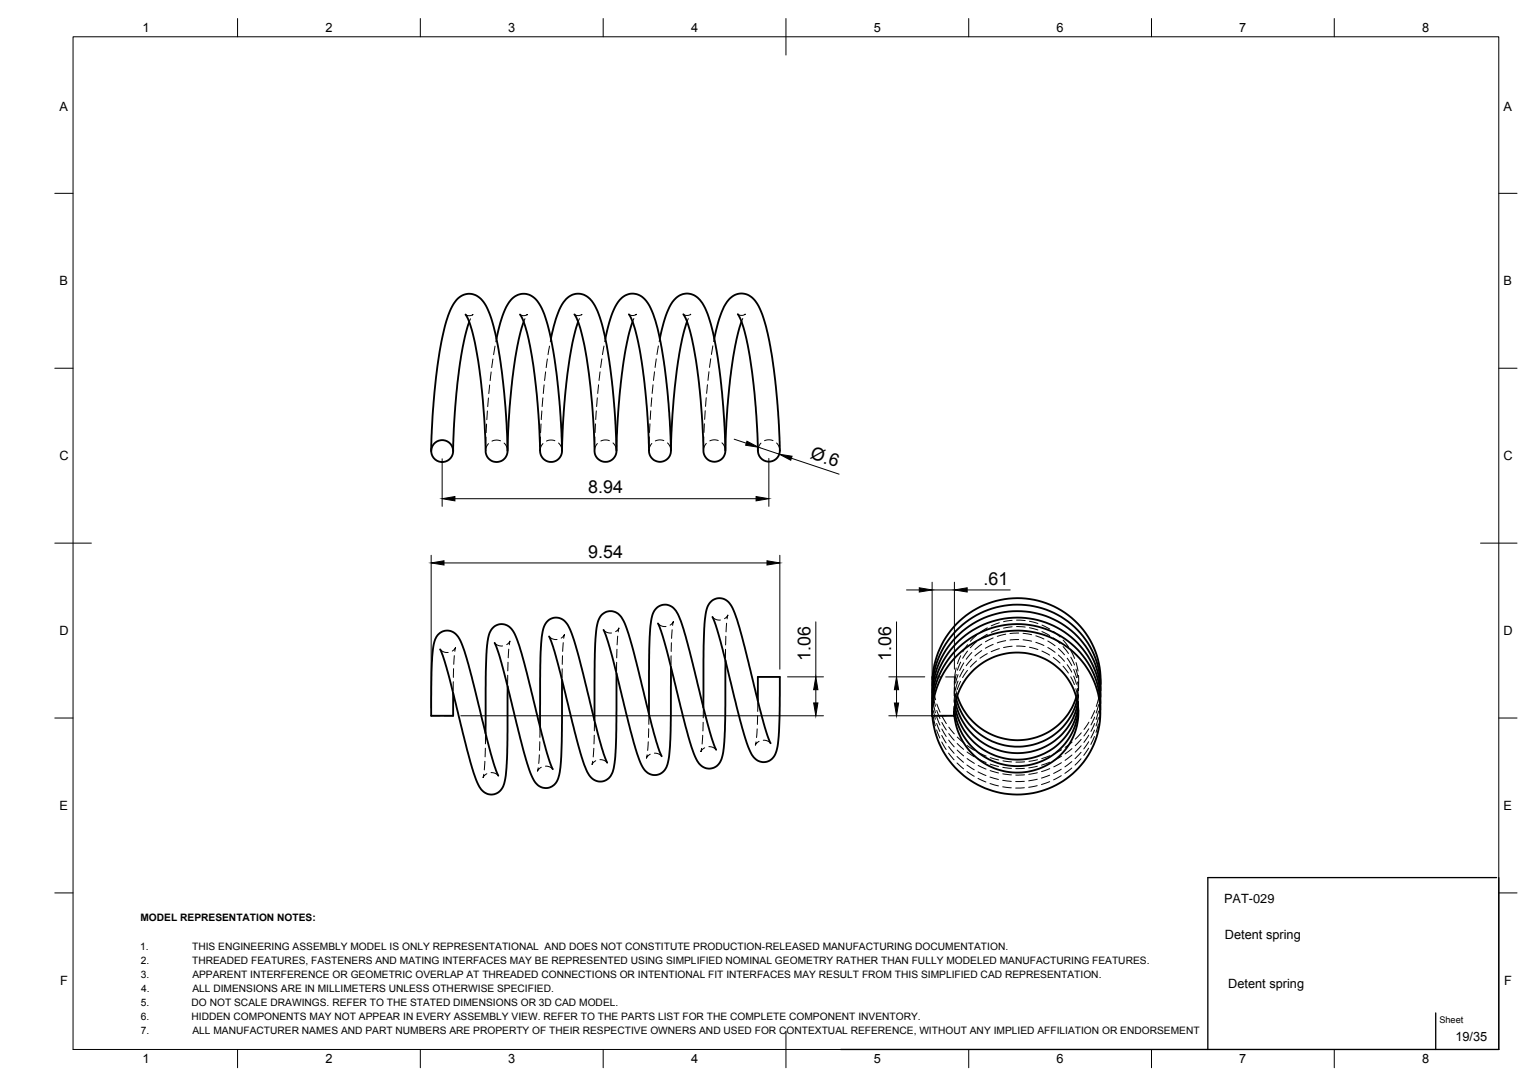
ISO-10303-21;
HEADER;
/* Generated by software containing ST-Developer
 * from STEP Tools, Inc. (www.steptools.com) 
 */

FILE_DESCRIPTION(
/* description */ ('Door-style hinge test fixture with detent'),
/* implementation_level */ '2;1');

FILE_NAME(
/* name */ 'Detent spring.step',
/* time_stamp */ '2026-10-28T03:24:57-07:00',
/* author */ (''),
/* organization */ (''),
/* preprocessor_version */ 'ST-DEVELOPER v20.2',
/* originating_system */ 'Autodesk Translation Framework v15.17.0.0',
/* authorisation */ '');

FILE_SCHEMA (('AUTOMOTIVE_DESIGN { 1 0 10303 214 3 1 1 }'));
ENDSEC;

DATA;
#10=MECHANICAL_DESIGN_GEOMETRIC_PRESENTATION_REPRESENTATION('',(#337),#9813);
#221=B_SPLINE_CURVE_WITH_KNOTS('',3,(#8567,#8568,#8569,#8570,#8571,#8572,
#8573,#8574,#8575,#8576,#8577,#8578,#8579,#8580,#8581,#8582,#8583,#8584,
#8585,#8586,#8587,#8588,#8589,#8590,#8591,#8592,#8593,#8594,#8595,#8596,
#8597,#8598,#8599,#8600,#8601,#8602,#8603,#8604,#8605,#8606,#8607,#8608,
#8609,#8610,#8611,#8612,#8613,#8614,#8615,#8616,#8617,#8618,#8619,#8620,
#8621,#8622,#8623,#8624,#8625,#8626,#8627,#8628,#8629,#8630,#8631),
 .UNSPECIFIED.,.F.,.F.,(4,1,1,1,1,1,1,1,1,1,1,1,1,1,1,1,1,1,1,1,1,1,1,1,
1,1,1,1,1,1,1,1,1,1,1,1,1,1,1,1,1,1,1,1,1,1,1,1,1,1,1,1,1,1,1,1,1,1,1,1,
1,1,4),(0.,0.0178571428571429,0.0357142857142857,0.0535714285714286,0.0714285714285714,
0.0892857142857143,0.107142857142857,0.125,0.142857142857143,0.158730158730159,
0.174603174603175,0.19047619047619,0.202380952380952,0.214285714285714,
0.226190476190476,0.238095238095238,0.25,0.261904761904762,0.273809523809524,
0.285714285714286,0.30952380952381,0.333333333333333,0.357142857142857,
0.380952380952381,0.404761904761905,0.428571428571429,0.446428571428571,
0.464285714285714,0.482142857142857,0.5,0.508928571428571,0.517857142857143,
0.535714285714286,0.553571428571429,0.571428571428571,0.589285714285714,
0.607142857142857,0.625,0.642857142857143,0.660714285714286,0.678571428571428,
0.696428571428571,0.714285714285714,0.738095238095238,0.75,0.761904761904762,
0.773809523809524,0.785714285714286,0.797619047619047,0.809523809523809,
0.821428571428571,0.833333333333333,0.845238095238095,0.857142857142857,
0.866071428571429,0.875,0.892857142857143,0.910714285714286,0.928571428571429,
0.946428571428571,0.964285714285714,0.982142857142857,1.),.UNSPECIFIED.);
#241=B_SPLINE_SURFACE_WITH_KNOTS('',3,3,((#7914,#7915,#7916,#7917,#7918,
#7919,#7920,#7921,#7922,#7923,#7924,#7925,#7926,#7927,#7928,#7929,#7930,
#7931,#7932,#7933,#7934,#7935,#7936,#7937,#7938,#7939,#7940,#7941,#7942,
#7943,#7944,#7945,#7946,#7947,#7948,#7949,#7950,#7951,#7952,#7953,#7954,
#7955,#7956,#7957,#7958,#7959,#7960,#7961,#7962,#7963,#7964,#7965,#7966,
#7967,#7968,#7969,#7970,#7971,#7972,#7973,#7974,#7975,#7976,#7977,#7978),
(#7979,#7980,#7981,#7982,#7983,#7984,#7985,#7986,#7987,#7988,#7989,#7990,
#7991,#7992,#7993,#7994,#7995,#7996,#7997,#7998,#7999,#8000,#8001,#8002,
#8003,#8004,#8005,#8006,#8007,#8008,#8009,#8010,#8011,#8012,#8013,#8014,
#8015,#8016,#8017,#8018,#8019,#8020,#8021,#8022,#8023,#8024,#8025,#8026,
#8027,#8028,#8029,#8030,#8031,#8032,#8033,#8034,#8035,#8036,#8037,#8038,
#8039,#8040,#8041,#8042,#8043),(#8044,#8045,#8046,#8047,#8048,#8049,#8050,
#8051,#8052,#8053,#8054,#8055,#8056,#8057,#8058,#8059,#8060,#8061,#8062,
#8063,#8064,#8065,#8066,#8067,#8068,#8069,#8070,#8071,#8072,#8073,#8074,
#8075,#8076,#8077,#8078,#8079,#8080,#8081,#8082,#8083,#8084,#8085,#8086,
#8087,#8088,#8089,#8090,#8091,#8092,#8093,#8094,#8095,#8096,#8097,#8098,
#8099,#8100,#8101,#8102,#8103,#8104,#8105,#8106,#8107,#8108),(#8109,#8110,
#8111,#8112,#8113,#8114,#8115,#8116,#8117,#8118,#8119,#8120,#8121,#8122,
#8123,#8124,#8125,#8126,#8127,#8128,#8129,#8130,#8131,#8132,#8133,#8134,
#8135,#8136,#8137,#8138,#8139,#8140,#8141,#8142,#8143,#8144,#8145,#8146,
#8147,#8148,#8149,#8150,#8151,#8152,#8153,#8154,#8155,#8156,#8157,#8158,
#8159,#8160,#8161,#8162,#8163,#8164,#8165,#8166,#8167,#8168,#8169,#8170,
#8171,#8172,#8173),(#8174,#8175,#8176,#8177,#8178,#8179,#8180,#8181,#8182,
#8183,#8184,#8185,#8186,#8187,#8188,#8189,#8190,#8191,#8192,#8193,#8194,
#8195,#8196,#8197,#8198,#8199,#8200,#8201,#8202,#8203,#8204,#8205,#8206,
#8207,#8208,#8209,#8210,#8211,#8212,#8213,#8214,#8215,#8216,#8217,#8218,
#8219,#8220,#8221,#8222,#8223,#8224,#8225,#8226,#8227,#8228,#8229,#8230,
#8231,#8232,#8233,#8234,#8235,#8236,#8237,#8238),(#8239,#8240,#8241,#8242,
#8243,#8244,#8245,#8246,#8247,#8248,#8249,#8250,#8251,#8252,#8253,#8254,
#8255,#8256,#8257,#8258,#8259,#8260,#8261,#8262,#8263,#8264,#8265,#8266,
#8267,#8268,#8269,#8270,#8271,#8272,#8273,#8274,#8275,#8276,#8277,#8278,
#8279,#8280,#8281,#8282,#8283,#8284,#8285,#8286,#8287,#8288,#8289,#8290,
#8291,#8292,#8293,#8294,#8295,#8296,#8297,#8298,#8299,#8300,#8301,#8302,
#8303),(#8304,#8305,#8306,#8307,#8308,#8309,#8310,#8311,#8312,#8313,#8314,
#8315,#8316,#8317,#8318,#8319,#8320,#8321,#8322,#8323,#8324,#8325,#8326,
#8327,#8328,#8329,#8330,#8331,#8332,#8333,#8334,#8335,#8336,#8337,#8338,
#8339,#8340,#8341,#8342,#8343,#8344,#8345,#8346,#8347,#8348,#8349,#8350,
#8351,#8352,#8353,#8354,#8355,#8356,#8357,#8358,#8359,#8360,#8361,#8362,
#8363,#8364,#8365,#8366,#8367,#8368),(#8369,#8370,#8371,#8372,#8373,#8374,
#8375,#8376,#8377,#8378,#8379,#8380,#8381,#8382,#8383,#8384,#8385,#8386,
#8387,#8388,#8389,#8390,#8391,#8392,#8393,#8394,#8395,#8396,#8397,#8398,
#8399,#8400,#8401,#8402,#8403,#8404,#8405,#8406,#8407,#8408,#8409,#8410,
#8411,#8412,#8413,#8414,#8415,#8416,#8417,#8418,#8419,#8420,#8421,#8422,
#8423,#8424,#8425,#8426,#8427,#8428,#8429,#8430,#8431,#8432,#8433),(#8434,
#8435,#8436,#8437,#8438,#8439,#8440,#8441,#8442,#8443,#8444,#8445,#8446,
#8447,#8448,#8449,#8450,#8451,#8452,#8453,#8454,#8455,#8456,#8457,#8458,
#8459,#8460,#8461,#8462,#8463,#8464,#8465,#8466,#8467,#8468,#8469,#8470,
#8471,#8472,#8473,#8474,#8475,#8476,#8477,#8478,#8479,#8480,#8481,#8482,
#8483,#8484,#8485,#8486,#8487,#8488,#8489,#8490,#8491,#8492,#8493,#8494,
#8495,#8496,#8497,#8498),(#8499,#8500,#8501,#8502,#8503,#8504,#8505,#8506,
#8507,#8508,#8509,#8510,#8511,#8512,#8513,#8514,#8515,#8516,#8517,#8518,
#8519,#8520,#8521,#8522,#8523,#8524,#8525,#8526,#8527,#8528,#8529,#8530,
#8531,#8532,#8533,#8534,#8535,#8536,#8537,#8538,#8539,#8540,#8541,#8542,
#8543,#8544,#8545,#8546,#8547,#8548,#8549,#8550,#8551,#8552,#8553,#8554,
#8555,#8556,#8557,#8558,#8559,#8560,#8561,#8562,#8563)),.UNSPECIFIED.,.T.,
 .F.,.F.,(4,1,1,1,1,1,1,4),(4,1,1,1,1,1,1,1,1,1,1,1,1,1,1,1,1,1,1,1,1,1,
1,1,1,1,1,1,1,1,1,1,1,1,1,1,1,1,1,1,1,1,1,1,1,1,1,1,1,1,1,1,1,1,1,1,1,1,
1,1,1,1,4),(-3.14159265358979,-2.24399475256414,-1.34639685153848,-0.448798950512828,
0.448798950512828,1.34639685153848,2.24399475256414,3.14159265358979),(0.,
0.0178571428571429,0.0357142857142857,0.0535714285714286,0.0714285714285714,
0.0892857142857143,0.107142857142857,0.125,0.142857142857143,0.158730158730159,
0.174603174603175,0.19047619047619,0.202380952380952,0.214285714285714,
0.226190476190476,0.238095238095238,0.25,0.261904761904762,0.273809523809524,
0.285714285714286,0.30952380952381,0.333333333333333,0.357142857142857,
0.380952380952381,0.404761904761905,0.428571428571429,0.446428571428571,
0.464285714285714,0.482142857142857,0.5,0.508928571428571,0.517857142857143,
0.535714285714286,0.553571428571429,0.571428571428571,0.589285714285714,
0.607142857142857,0.625,0.642857142857143,0.660714285714286,0.678571428571428,
0.696428571428571,0.714285714285714,0.738095238095238,0.75,0.761904761904762,
0.773809523809524,0.785714285714286,0.797619047619047,0.809523809523809,
0.821428571428571,0.833333333333333,0.845238095238095,0.857142857142857,
0.866071428571429,0.875,0.892857142857143,0.910714285714286,0.928571428571429,
0.946428571428571,0.964285714285714,0.982142857142857,1.),.UNSPECIFIED.);
#274=SHAPE_REPRESENTATION_RELATIONSHIP('SRR','None',#9951,#305);
#305=ADVANCED_BREP_SHAPE_REPRESENTATION('',(#377),#9794);
#337=STYLED_ITEM('',(#10183),#377);
#377=MANIFOLD_SOLID_BREP('Body1',#4768);
#578=PLANE('',#5393);
#579=PLANE('',#5394);
#790=FACE_OUTER_BOUND('',#1141,.T.);
#791=FACE_OUTER_BOUND('',#1142,.T.);
#792=FACE_OUTER_BOUND('',#1143,.T.);
#1141=EDGE_LOOP('',(#3773,#3774,#3775,#3776));
#1142=EDGE_LOOP('',(#3777));
#1143=EDGE_LOOP('',(#3778));
#2083=CIRCLE('',#5391,0.03);
#2084=CIRCLE('',#5392,0.03);
#2411=VERTEX_POINT('',#8564);
#2412=VERTEX_POINT('',#8566);
#2903=EDGE_CURVE('',#2411,#2411,#2083,.T.);
#2904=EDGE_CURVE('',#2411,#2412,#221,.T.);
#2905=EDGE_CURVE('',#2412,#2412,#2084,.T.);
#3773=ORIENTED_EDGE('',*,*,#2903,.T.);
#3774=ORIENTED_EDGE('',*,*,#2904,.T.);
#3775=ORIENTED_EDGE('',*,*,#2905,.F.);
#3776=ORIENTED_EDGE('',*,*,#2904,.F.);
#3777=ORIENTED_EDGE('',*,*,#2905,.T.);
#3778=ORIENTED_EDGE('',*,*,#2903,.F.);
#4595=ADVANCED_FACE('',(#790),#241,.T.);
#4596=ADVANCED_FACE('',(#791),#578,.T.);
#4597=ADVANCED_FACE('',(#792),#579,.F.);
#4768=CLOSED_SHELL('',(#4595,#4596,#4597));
#5390=AXIS2_PLACEMENT_3D('',#7913,#6429,#6430);
#5391=AXIS2_PLACEMENT_3D('',#8565,#6431,#6432);
#5392=AXIS2_PLACEMENT_3D('',#8632,#6433,#6434);
#5393=AXIS2_PLACEMENT_3D('',#8633,#6435,#6436);
#5394=AXIS2_PLACEMENT_3D('',#8634,#6437,#6438);
#6429=DIRECTION('axis',(0.,0.,1.));
#6430=DIRECTION('refdir',(1.,0.,0.));
#6431=DIRECTION('center_axis',(-0.000133970394124395,-0.118176177591672,
0.992992634968536));
#6432=DIRECTION('ref_axis',(1.59438332031483E-5,-0.992992644005897,-0.118176176516135));
#6433=DIRECTION('center_axis',(0.000133970209996934,-0.118176177452328,
0.992992634985144));
#6434=DIRECTION('ref_axis',(0.970349186816215,0.240028974349624,0.0284349629466645));
#6435=DIRECTION('center_axis',(0.000133970209996934,-0.118176177452328,
0.992992634985144));
#6436=DIRECTION('ref_axis',(0.970349186816215,0.240028974349624,0.0284349629466645));
#6437=DIRECTION('center_axis',(-0.000133970394124395,-0.118176177591672,
0.992992634968536));
#6438=DIRECTION('ref_axis',(1.59438332031483E-5,-0.992992644005897,-0.118176176516135));
#7913=CARTESIAN_POINT('',(0.,0.,0.));
#7914=CARTESIAN_POINT('Ctrl Pts',(0.199999521685004,-2.62021022067982,7.20354528529548));
#7915=CARTESIAN_POINT('Ctrl Pts',(0.19999343949118,-2.6255753643916,7.24862669087077));
#7916=CARTESIAN_POINT('Ctrl Pts',(0.168615691452697,-2.63634781999191,7.33868016798294));
#7917=CARTESIAN_POINT('Ctrl Pts',(0.0459616996448183,-2.65270477799173,
7.41618164971903));
#7918=CARTESIAN_POINT('Ctrl Pts',(-0.0998469869656992,-2.66924595959392,
7.39996507729611));
#7919=CARTESIAN_POINT('Ctrl Pts',(-0.204936181985623,-2.68597304189578,
7.29527847685269));
#7920=CARTESIAN_POINT('Ctrl Pts',(-0.221986969755699,-2.7028797483455,7.14628505326925));
#7921=CARTESIAN_POINT('Ctrl Pts',(-0.141631327334848,-2.71996166380803,
7.01788664502262));
#7922=CARTESIAN_POINT('Ctrl Pts',(0.00270481241442627,-2.73721192504324,
6.96708134679183));
#7923=CARTESIAN_POINT('Ctrl Pts',(0.143039113459417,-2.75397833948373,7.01603761180454));
#7924=CARTESIAN_POINT('Ctrl Pts',(0.223330027417085,-2.77023316539608,7.13370506584288));
#7925=CARTESIAN_POINT('Ctrl Pts',(0.223609433092684,-2.7859516486779,7.2713911725354));
#7926=CARTESIAN_POINT('Ctrl Pts',(0.152101468687107,-2.80045790761646,7.37648984952004));
#7927=CARTESIAN_POINT('Ctrl Pts',(0.0493840180807327,-2.81371750007274,
7.42583309513969));
#7928=CARTESIAN_POINT('Ctrl Pts',(-0.0535656424988985,-2.82570326133932,
7.42596307871198));
#7929=CARTESIAN_POINT('Ctrl Pts',(-0.146731811694293,-2.83773755003964,
7.38108373553243));
#7930=CARTESIAN_POINT('Ctrl Pts',(-0.211512387655128,-2.8498166397957,7.29998894076038));
#7931=CARTESIAN_POINT('Ctrl Pts',(-0.234672692510252,-2.86193666288461,
7.19851881716116));
#7932=CARTESIAN_POINT('Ctrl Pts',(-0.211502078818359,-2.87409363541626,
7.09651570260184));
#7933=CARTESIAN_POINT('Ctrl Pts',(-0.146175031667225,-2.88628349462379,
7.01496045942807));
#7934=CARTESIAN_POINT('Ctrl Pts',(-0.0201759406699065,-2.90257490033143,
6.95334279019282));
#7935=CARTESIAN_POINT('Ctrl Pts',(0.164048433167981,-2.92300029227989,6.99488705015939));
#7936=CARTESIAN_POINT('Ctrl Pts',(0.263212640482471,-2.94757377707087,7.20034626829039));
#7937=CARTESIAN_POINT('Ctrl Pts',(0.16413428164115,-2.9721746956776,7.40571604889496));
#7938=CARTESIAN_POINT('Ctrl Pts',(-0.0580809020736254,-2.99676718133414,
7.45651943873815));
#7939=CARTESIAN_POINT('Ctrl Pts',(-0.236127517621773,-3.02131545740765,
7.31427023254914));
#7940=CARTESIAN_POINT('Ctrl Pts',(-0.235623291843773,-3.04374517395574,
7.10674242176483));
#7941=CARTESIAN_POINT('Ctrl Pts',(-0.107269644782094,-3.06405280900675,
6.97972425972366));
#7942=CARTESIAN_POINT('Ctrl Pts',(0.0527757922260714,-3.08225163138773,
6.96159979137369));
#7943=CARTESIAN_POINT('Ctrl Pts',(0.188726377923501,-3.10035885514916,7.04734634676648));
#7944=CARTESIAN_POINT('Ctrl Pts',(0.232341637226282,-3.11536108595312,7.17289318656827));
#7945=CARTESIAN_POINT('Ctrl Pts',(0.215074929637344,-3.12730445561105,7.27290788199928));
#7946=CARTESIAN_POINT('Ctrl Pts',(0.166334604203376,-3.13920694864625,7.3615533699487));
#7947=CARTESIAN_POINT('Ctrl Pts',(0.0552567235661542,-3.1540048293497,7.43128948802867));
#7948=CARTESIAN_POINT('Ctrl Pts',(-0.100043793704833,-3.17162317434127,
7.4135433615447));
#7949=CARTESIAN_POINT('Ctrl Pts',(-0.209398878386583,-3.18909256344761,
7.30384381469642));
#7950=CARTESIAN_POINT('Ctrl Pts',(-0.226357160076232,-3.20640410002376,
7.15124619930781));
#7951=CARTESIAN_POINT('Ctrl Pts',(-0.145244888291477,-3.22354989628281,
7.02263774678675));
#7952=CARTESIAN_POINT('Ctrl Pts',(-0.00307739889558997,-3.24052311289208,
6.9731562179116));
#7953=CARTESIAN_POINT('Ctrl Pts',(0.137388780060693,-3.25731801286151,7.02262233145429));
#7954=CARTESIAN_POINT('Ctrl Pts',(0.215568012201749,-3.27392998789316,7.14745036721));
#7955=CARTESIAN_POINT('Ctrl Pts',(0.199056669422034,-3.29035561704227,7.29224338602279));
#7956=CARTESIAN_POINT('Ctrl Pts',(0.0972442378117871,-3.30659260084323,
7.39359267072072));
#7957=CARTESIAN_POINT('Ctrl Pts',(-0.0606078656788346,-3.32442299860284,
7.41159207397961));
#7958=CARTESIAN_POINT('Ctrl Pts',(-0.174349434794334,-3.34024917344643,
7.3202399790036));
#7959=CARTESIAN_POINT('Ctrl Pts',(-0.200242071600934,-3.35415023112003,
7.20325404432313));
#7960=CARTESIAN_POINT('Ctrl Pts',(-0.18063258547865,-3.36449358017806,7.11681410663695));
#7961=CARTESIAN_POINT('Ctrl Pts',(-0.125490051337177,-3.37475550369447,
7.04788845684967));
#7962=CARTESIAN_POINT('Ctrl Pts',(-0.0466957223057233,-3.38493729013136,
7.00998942647324));
#7963=CARTESIAN_POINT('Ctrl Pts',(0.0401186427931674,-3.39504044724382,
7.01009457046437));
#7964=CARTESIAN_POINT('Ctrl Pts',(0.117713403951327,-3.40506669595631,7.04749596858794));
#7965=CARTESIAN_POINT('Ctrl Pts',(0.170930387597076,-3.41501799177983,7.11440539415709));
#7966=CARTESIAN_POINT('Ctrl Pts',(0.18979238088286,-3.42489648282701,7.1971524208448));
#7967=CARTESIAN_POINT('Ctrl Pts',(0.17093827709221,-3.43470453492267,7.2792766512254));
#7968=CARTESIAN_POINT('Ctrl Pts',(0.123087817102158,-3.44363304446436,7.33923456804198));
#7969=CARTESIAN_POINT('Ctrl Pts',(0.0630389653927127,-3.45170235370222,
7.37229315652779));
#7970=CARTESIAN_POINT('Ctrl Pts',(-0.0177036729288225,-3.46133839204526,
7.38615351281265));
#7971=CARTESIAN_POINT('Ctrl Pts',(-0.11772305137169,-3.47329787855213,7.35109019812551));
#7972=CARTESIAN_POINT('Ctrl Pts',(-0.184714685581635,-3.48752403008714,
7.24410703240861));
#7973=CARTESIAN_POINT('Ctrl Pts',(-0.17053859750796,-3.50163575663314,7.11977423357787));
#7974=CARTESIAN_POINT('Ctrl Pts',(-0.082587996452088,-3.51564730527911,
7.03201669890537));
#7975=CARTESIAN_POINT('Ctrl Pts',(0.0401074098738201,-3.52956782204744,
7.0182572369454));
#7976=CARTESIAN_POINT('Ctrl Pts',(0.144033604536224,-3.54341977713357,7.08377705773452));
#7977=CARTESIAN_POINT('Ctrl Pts',(0.170884312908661,-3.55260377562906,7.16051919899628));
#7978=CARTESIAN_POINT('Ctrl Pts',(0.170889524395514,-3.55720086923049,7.1991469511116));
#7979=CARTESIAN_POINT('Ctrl Pts',(0.191023542756439,-2.62021022067982,7.20354407429412));
#7980=CARTESIAN_POINT('Ctrl Pts',(0.191017726414002,-2.62534085511048,7.24665498129917));
#7981=CARTESIAN_POINT('Ctrl Pts',(0.161033850394857,-2.63563485658156,7.33273947644214));
#7982=CARTESIAN_POINT('Ctrl Pts',(0.0436799375629447,-2.6512854138931,7.40693000436112));
#7983=CARTESIAN_POINT('Ctrl Pts',(-0.0959987808218971,-2.66712696375714,
7.39142052099388));
#7984=CARTESIAN_POINT('Ctrl Pts',(-0.196829905250034,-2.68316922567495,
7.29102743103875));
#7985=CARTESIAN_POINT('Ctrl Pts',(-0.213252255362172,-2.69940855979398,
7.14788433221334));
#7986=CARTESIAN_POINT('Ctrl Pts',(-0.135952056419508,-2.71584543096616,
7.0242793563294));
#7987=CARTESIAN_POINT('Ctrl Pts',(0.00322439729343584,-2.73247671681477,
6.97523297281595));
#7988=CARTESIAN_POINT('Ctrl Pts',(0.138869091438245,-2.74867593022619,7.02249383745227));
#7989=CARTESIAN_POINT('Ctrl Pts',(0.216674071017294,-2.76441519194789,7.13643570930967));
#7990=CARTESIAN_POINT('Ctrl Pts',(0.216990443986426,-2.77967065524482,7.27008142439094));
#7991=CARTESIAN_POINT('Ctrl Pts',(0.147461738971512,-2.79377910905693,7.37235184002062));
#7992=CARTESIAN_POINT('Ctrl Pts',(0.047333450735047,-2.80670380678563,7.42047652131588));
#7993=CARTESIAN_POINT('Ctrl Pts',(-0.0532106536911018,-2.81840737559959,
7.4206256558615));
#7994=CARTESIAN_POINT('Ctrl Pts',(-0.144378744511407,-2.83018047137138,
7.37673185790055));
#7995=CARTESIAN_POINT('Ctrl Pts',(-0.207902064816201,-2.84201938593495,
7.29724909461857));
#7996=CARTESIAN_POINT('Ctrl Pts',(-0.230670002371674,-2.85392183859013,
7.19758944399363));
#7997=CARTESIAN_POINT('Ctrl Pts',(-0.207893335338729,-2.86588164249669,
7.0972028957719));
#7998=CARTESIAN_POINT('Ctrl Pts',(-0.143487364744061,-2.87790004133283,
7.01676930123252));
#7999=CARTESIAN_POINT('Ctrl Pts',(-0.0190193226663081,-2.89399389208917,
6.95585884391441));
#8000=CARTESIAN_POINT('Ctrl Pts',(0.163586328894419,-2.91422968067412,6.99687105352309));
#8001=CARTESIAN_POINT('Ctrl Pts',(0.262456471900163,-2.9386767814229,7.20122686982788));
#8002=CARTESIAN_POINT('Ctrl Pts',(0.16364689697854,-2.96325138569098,7.40652598693401));
#8003=CARTESIAN_POINT('Ctrl Pts',(-0.059251333627089,-2.98791913148238,
7.45770124310656));
#8004=CARTESIAN_POINT('Ctrl Pts',(-0.238744875888964,-3.01264249790562,
7.31456854455266));
#8005=CARTESIAN_POINT('Ctrl Pts',(-0.238414861081409,-3.03532370670177,
7.1046723413934));
#8006=CARTESIAN_POINT('Ctrl Pts',(-0.108219790599525,-3.05592692071135,
6.97569591466389));
#8007=CARTESIAN_POINT('Ctrl Pts',(0.0546507861677333,-3.07444227191367,
6.95717854257545));
#8008=CARTESIAN_POINT('Ctrl Pts',(0.193437408460763,-3.09291982793468,7.04462472677658));
#8009=CARTESIAN_POINT('Ctrl Pts',(0.238122848764674,-3.10826703109889,7.17307568347903));
#8010=CARTESIAN_POINT('Ctrl Pts',(0.220429833499831,-3.12051104548578,7.2756216678726));
#8011=CARTESIAN_POINT('Ctrl Pts',(0.170406454940412,-3.13272858443559,7.36662390053473));
#8012=CARTESIAN_POINT('Ctrl Pts',(0.056200071240455,-3.14794419657849,7.43838646727187));
#8013=CARTESIAN_POINT('Ctrl Pts',(-0.103895504850653,-3.16610350899751,
7.42015451305419));
#8014=CARTESIAN_POINT('Ctrl Pts',(-0.216908103553831,-3.18414862458417,
7.30686416228629));
#8015=CARTESIAN_POINT('Ctrl Pts',(-0.234513691775253,-3.20206759837303,
7.14890287443755));
#8016=CARTESIAN_POINT('Ctrl Pts',(-0.150429627901186,-3.2198483950201,7.01549612364992));
#8017=CARTESIAN_POINT('Ctrl Pts',(-0.00275052944868849,-3.23748023207103,
6.96405310813854));
#8018=CARTESIAN_POINT('Ctrl Pts',(0.143402720749719,-3.2549531655216,7.01548469083049));
#8019=CARTESIAN_POINT('Ctrl Pts',(0.224869691209636,-3.27225819798112,7.14550628408959));
#8020=CARTESIAN_POINT('Ctrl Pts',(0.207674446226838,-3.2893875862004,7.2965024724066));
#8021=CARTESIAN_POINT('Ctrl Pts',(0.101426890655383,-3.30633493427357,7.40228966269414));
#8022=CARTESIAN_POINT('Ctrl Pts',(-0.0634150898376773,-3.32495614129161,
7.4210979000742));
#8023=CARTESIAN_POINT('Ctrl Pts',(-0.1822359591826,-3.34149060327876,7.32567014640293));
#8024=CARTESIAN_POINT('Ctrl Pts',(-0.209280485902103,-3.35601236711325,
7.20346528253749));
#8025=CARTESIAN_POINT('Ctrl Pts',(-0.188795825646846,-3.36681636246986,
7.11318643013913));
#8026=CARTESIAN_POINT('Ctrl Pts',(-0.131216307204934,-3.37753199733383,
7.04122143073785));
#8027=CARTESIAN_POINT('Ctrl Pts',(-0.048975801731852,-3.3881599612999,7.00167277093901));
#8028=CARTESIAN_POINT('Ctrl Pts',(0.0415822516777477,-3.39869985613274,
7.00178871033236));
#8029=CARTESIAN_POINT('Ctrl Pts',(0.122464106224022,-3.40915267810657,7.04078440402212));
#8030=CARTESIAN_POINT('Ctrl Pts',(0.177886120551665,-3.41951877896738,7.11047882697577));
#8031=CARTESIAN_POINT('Ctrl Pts',(0.197502916828992,-3.42979927641084,7.19658381053113));
#8032=CARTESIAN_POINT('Ctrl Pts',(0.177896449457243,-3.43999561916638,7.28194224811453));
#8033=CARTESIAN_POINT('Ctrl Pts',(0.128212743394908,-3.44926556361253,7.34417843697285));
#8034=CARTESIAN_POINT('Ctrl Pts',(0.0659471883228922,-3.45763455664724,
7.37845138672491));
#8035=CARTESIAN_POINT('Ctrl Pts',(-0.0176843848898256,-3.46761643973737,
7.39279899859123));
#8036=CARTESIAN_POINT('Ctrl Pts',(-0.121083708756642,-3.47998778018346,
7.35650173270899));
#8037=CARTESIAN_POINT('Ctrl Pts',(-0.190111930497616,-3.49466307862108,
7.24614193421259));
#8038=CARTESIAN_POINT('Ctrl Pts',(-0.175463764144624,-3.50917928747668,
7.11830222206023));
#8039=CARTESIAN_POINT('Ctrl Pts',(-0.0852554106795787,-3.52354649168734,
7.02839732944465));
#8040=CARTESIAN_POINT('Ctrl Pts',(0.0401061072486938,-3.53777296100086,
7.01441443337408));
#8041=CARTESIAN_POINT('Ctrl Pts',(0.145858454765231,-3.55187732457476,7.0811740864261));
#8042=CARTESIAN_POINT('Ctrl Pts',(0.17305380815376,-3.56119542074233,7.1590096425235));
#8043=CARTESIAN_POINT('Ctrl Pts',(0.173059084396458,-3.56584963598494,7.19811736759295));
#8044=CARTESIAN_POINT('Ctrl Pts',(0.173158501738058,-2.62873184854516,7.20252750402056));
#8045=CARTESIAN_POINT('Ctrl Pts',(0.173153218829459,-2.63339193743202,7.2416845831989));
#8046=CARTESIAN_POINT('Ctrl Pts',(0.145938970756177,-2.64272474633487,7.31968447296958));
#8047=CARTESIAN_POINT('Ctrl Pts',(0.0397348763892528,-2.65689026062815,
7.38679369226741));
#8048=CARTESIAN_POINT('Ctrl Pts',(-0.0864890400134375,-2.67120973124552,
7.37274979393911));
#8049=CARTESIAN_POINT('Ctrl Pts',(-0.177560438111068,-2.68570416834132,
7.28207185920492));
#8050=CARTESIAN_POINT('Ctrl Pts',(-0.192407596533418,-2.70037922212494,
7.15275928313263));
#8051=CARTESIAN_POINT('Ctrl Pts',(-0.122540417469413,-2.71524574150998,
7.0409920671935));
#8052=CARTESIAN_POINT('Ctrl Pts',(0.00346341303810412,-2.73031050711819,
6.99654562940632));
#8053=CARTESIAN_POINT('Ctrl Pts',(0.126554930146189,-2.74501481989148,7.03938106158892));
#8054=CARTESIAN_POINT('Ctrl Pts',(0.197363865868405,-2.75933707765723,7.14299597376079));
#8055=CARTESIAN_POINT('Ctrl Pts',(0.197704056060021,-2.77325401319431,7.26489099146508));
#8056=CARTESIAN_POINT('Ctrl Pts',(0.134130381062669,-2.786168336898,7.35849624306076));
#8057=CARTESIAN_POINT('Ctrl Pts',(0.0422460255745021,-2.79803276136078,
7.40269519912191));
#8058=CARTESIAN_POINT('Ctrl Pts',(-0.0502919619965319,-2.8088075022445,
7.40285907057282));
#8059=CARTESIAN_POINT('Ctrl Pts',(-0.134469523268098,-2.81967842050119,
7.36236888554382));
#8060=CARTESIAN_POINT('Ctrl Pts',(-0.193322485979024,-2.83064537823505,
7.28878115409414));
#8061=CARTESIAN_POINT('Ctrl Pts',(-0.214513633921132,-2.84170727748237,
7.19618893172989));
#8062=CARTESIAN_POINT('Ctrl Pts',(-0.193316277704633,-2.85286429839084,
7.10257534531843));
#8063=CARTESIAN_POINT('Ctrl Pts',(-0.133070873823438,-2.86411323797119,
7.0272822312058));
#8064=CARTESIAN_POINT('Ctrl Pts',(-0.0162062490412889,-2.87923391733063,
6.97002261633703));
#8065=CARTESIAN_POINT('Ctrl Pts',(0.156368886155166,-2.89836026042033,7.00846997516318));
#8066=CARTESIAN_POINT('Ctrl Pts',(0.250905090253854,-2.9216527068464,7.20291604024908));
#8067=CARTESIAN_POINT('Ctrl Pts',(0.156382586273267,-2.94526590871319,7.40029658879584));
#8068=CARTESIAN_POINT('Ctrl Pts',(-0.0594801303014584,-2.96917467862821,
7.45031261861394));
#8069=CARTESIAN_POINT('Ctrl Pts',(-0.235239905615142,-2.99335132894538,
7.31075364916488));
#8070=CARTESIAN_POINT('Ctrl Pts',(-0.235324261158338,-3.01572980435851,
7.10370529224427));
#8071=CARTESIAN_POINT('Ctrl Pts',(-0.10602170037884,-3.03622281987395,6.9752854815943));
#8072=CARTESIAN_POINT('Ctrl Pts',(0.0570006024249987,-3.05476604528251,
6.95657099108577));
#8073=CARTESIAN_POINT('Ctrl Pts',(0.196978986837661,-3.07339085238332,7.04453594814324));
#8074=CARTESIAN_POINT('Ctrl Pts',(0.242467752552828,-3.08896870185106,7.1748237890863));
#8075=CARTESIAN_POINT('Ctrl Pts',(0.224455215333573,-3.10145518627921,7.27939935476355));
#8076=CARTESIAN_POINT('Ctrl Pts',(0.17331013027485,-3.11395563571474,7.37250667012694));
#8077=CARTESIAN_POINT('Ctrl Pts',(0.0559775593867093,-3.12960297019709,
7.44641139018859));
#8078=CARTESIAN_POINT('Ctrl Pts',(-0.109693476081705,-3.14839546460465,
7.42772920012961));
#8079=CARTESIAN_POINT('Ctrl Pts',(-0.227486258030471,-3.16718695551515,
7.30989707575346));
#8080=CARTESIAN_POINT('Ctrl Pts',(-0.246098856844244,-3.18595987633661,
7.14444836244404));
#8081=CARTESIAN_POINT('Ctrl Pts',(-0.157640602442323,-3.2046971614539,7.00379198862032));
#8082=CARTESIAN_POINT('Ctrl Pts',(-0.00120601544693738,-3.22338180286804,
6.9491324800669));
#8083=CARTESIAN_POINT('Ctrl Pts',(0.154546474484069,-3.24199717653129,7.00378599134579));
#8084=CARTESIAN_POINT('Ctrl Pts',(0.241897815202096,-3.26052712642461,7.14293476115058));
#8085=CARTESIAN_POINT('Ctrl Pts',(0.223524906976926,-3.27895597756738,7.30540511372487));
#8086=CARTESIAN_POINT('Ctrl Pts',(0.108790492948344,-3.29726854793425,7.41980440638438));
#8087=CARTESIAN_POINT('Ctrl Pts',(-0.0700533440103121,-3.31747119125551,
7.44034864847014));
#8088=CARTESIAN_POINT('Ctrl Pts',(-0.199623057501188,-3.33548579374738,
7.33648540438074));
#8089=CARTESIAN_POINT('Ctrl Pts',(-0.229221414974038,-3.35135671295434,
7.20291396417937));
#8090=CARTESIAN_POINT('Ctrl Pts',(-0.206809680372079,-3.36318519045383,
7.10405847819106));
#8091=CARTESIAN_POINT('Ctrl Pts',(-0.143675377283367,-3.37493610128364,
7.02511964802601));
#8092=CARTESIAN_POINT('Ctrl Pts',(-0.0533626365384458,-3.38660622159859,
6.98167021818281));
#8093=CARTESIAN_POINT('Ctrl Pts',(0.046205156976151,-3.39819313055781,6.98178625579333));
#8094=CARTESIAN_POINT('Ctrl Pts',(0.135218488600369,-3.40969412427728,7.02469031539363));
#8095=CARTESIAN_POINT('Ctrl Pts',(0.196251716945606,-3.42110716597797,7.10143474403484));
#8096=CARTESIAN_POINT('Ctrl Pts',(0.217865285391825,-3.4324301939502,7.1962892325178));
#8097=CARTESIAN_POINT('Ctrl Pts',(0.196260535910131,-3.44366140556578,7.29033280776571));
#8098=CARTESIAN_POINT('Ctrl Pts',(0.141526130922779,-3.45387157509335,7.35889127434652));
#8099=CARTESIAN_POINT('Ctrl Pts',(0.0729583886246232,-3.4630842452824,7.39662788506617));
#8100=CARTESIAN_POINT('Ctrl Pts',(-0.0190940690797755,-3.47406867882678,
7.41241609379824));
#8101=CARTESIAN_POINT('Ctrl Pts',(-0.132779160970955,-3.48766247485799,
7.37247540729533));
#8102=CARTESIAN_POINT('Ctrl Pts',(-0.208489105531237,-3.50375946110311,
7.25133738069355));
#8103=CARTESIAN_POINT('Ctrl Pts',(-0.192394326071967,-3.519638321504,7.11142720311936));
#8104=CARTESIAN_POINT('Ctrl Pts',(-0.0939403593005316,-3.53530277168423,
7.01341338007167));
#8105=CARTESIAN_POINT('Ctrl Pts',(0.0422605125078274,-3.55075075526385,
6.99832278160776));
#8106=CARTESIAN_POINT('Ctrl Pts',(0.1565440859987,-3.56599599233585,7.07060828215171));
#8107=CARTESIAN_POINT('Ctrl Pts',(0.185698876792587,-3.57601155541678,7.15436510947656));
#8108=CARTESIAN_POINT('Ctrl Pts',(0.185704536106873,-3.58100368112599,7.19631217672005));
#8109=CARTESIAN_POINT('Ctrl Pts',(0.166525366620545,-2.65758658420228,7.19909260340903));
#8110=CARTESIAN_POINT('Ctrl Pts',(0.166520289008348,-2.66206557976378,7.23672801940631));
#8111=CARTESIAN_POINT('Ctrl Pts',(0.140348275753376,-2.67098879281991,7.31126270005341));
#8112=CARTESIAN_POINT('Ctrl Pts',(0.0399774791194812,-2.68435583849075,
7.37438039593517));
#8113=CARTESIAN_POINT('Ctrl Pts',(-0.0776574996962614,-2.69770347508532,
7.36105620850106));
#8114=CARTESIAN_POINT('Ctrl Pts',(-0.161408766434036,-2.71105687135119,
7.27734776640516));
#8115=CARTESIAN_POINT('Ctrl Pts',(-0.174728238572193,-2.72442979432405,
7.15947416895345));
#8116=CARTESIAN_POINT('Ctrl Pts',(-0.111526458500605,-2.73784095508408,
7.05873826484987));
#8117=CARTESIAN_POINT('Ctrl Pts',(0.00117829704477278,-2.75130656740219,
7.01917259019172));
#8118=CARTESIAN_POINT('Ctrl Pts',(0.11026863481546,-2.7643421103719,7.05729331555389));
#8119=CARTESIAN_POINT('Ctrl Pts',(0.172542463585331,-2.77695269446299,7.14859557088421));
#8120=CARTESIAN_POINT('Ctrl Pts',(0.172758419267171,-2.78913933013576,7.25534594832492));
#8121=CARTESIAN_POINT('Ctrl Pts',(0.117297375174102,-2.80039298929176,7.33689338067046));
#8122=CARTESIAN_POINT('Ctrl Pts',(0.0374793460091744,-2.81069732757045,
7.37525827577019));
#8123=CARTESIAN_POINT('Ctrl Pts',(-0.0426999334578007,-2.82003179746841,
7.37538143917469));
#8124=CARTESIAN_POINT('Ctrl Pts',(-0.115480105067975,-2.82943089377101,
7.34035492146379));
#8125=CARTESIAN_POINT('Ctrl Pts',(-0.166283399534618,-2.8388982290778,7.2768148162638));
#8126=CARTESIAN_POINT('Ctrl Pts',(-0.184550847892414,-2.84843746708543,
7.19695788907849));
#8127=CARTESIAN_POINT('Ctrl Pts',(-0.166278739115269,-2.85805148397594,
7.11627641094483));
#8128=CARTESIAN_POINT('Ctrl Pts',(-0.11436157509869,-2.86774415878459,7.05139195278408));
#8129=CARTESIAN_POINT('Ctrl Pts',(-0.0136373605432596,-2.88077580648601,
7.00203726516335));
#8130=CARTESIAN_POINT('Ctrl Pts',(0.135270491135525,-2.8972745142599,7.03513970278866));
#8131=CARTESIAN_POINT('Ctrl Pts',(0.217212305752653,-2.91742718851122,7.20332132024231));
#8132=CARTESIAN_POINT('Ctrl Pts',(0.135257996783122,-2.93794808980581,7.37497192443284));
#8133=CARTESIAN_POINT('Ctrl Pts',(-0.0533876532778471,-2.9588476861815,
7.41897307812886));
#8134=CARTESIAN_POINT('Ctrl Pts',(-0.208357363305794,-2.98013180670875,
7.29637221500731));
#8135=CARTESIAN_POINT('Ctrl Pts',(-0.208783521385516,-2.99999644346923,
7.1125597718962));
#8136=CARTESIAN_POINT('Ctrl Pts',(-0.0932051793686978,-3.01833445242994,
6.99745969229246));
#8137=CARTESIAN_POINT('Ctrl Pts',(0.0537644028633427,-3.03505132869382,
6.98040447259593));
#8138=CARTESIAN_POINT('Ctrl Pts',(0.181096825444236,-3.05197751615123,7.06017345938295));
#8139=CARTESIAN_POINT('Ctrl Pts',(0.222956282771945,-3.06625169664934,7.17952184368757));
#8140=CARTESIAN_POINT('Ctrl Pts',(0.206375060569474,-3.07776961978831,7.27600523510941));
#8141=CARTESIAN_POINT('Ctrl Pts',(0.159022777496631,-3.08935174812889,7.36228595692239));
#8142=CARTESIAN_POINT('Ctrl Pts',(0.049676708892268,-3.10394701180979,7.43139250849058));
#8143=CARTESIAN_POINT('Ctrl Pts',(-0.106345964297192,-3.12164088568468,
7.41405454588476));
#8144=CARTESIAN_POINT('Ctrl Pts',(-0.218508477592453,-3.13950380517162,
7.30222030391762));
#8145=CARTESIAN_POINT('Ctrl Pts',(-0.236640596317295,-3.15752444745288,
7.14342530883726));
#8146=CARTESIAN_POINT('Ctrl Pts',(-0.151108234377237,-3.17569037824872,
7.00690875886963));
#8147=CARTESIAN_POINT('Ctrl Pts',(0.0020000497825991,-3.19398828187494,
6.95311663906165));
#8148=CARTESIAN_POINT('Ctrl Pts',(0.156175162605377,-3.2124039849716,7.00692181511878));
#8149=CARTESIAN_POINT('Ctrl Pts',(0.243712267918876,-3.23092257241902,7.14582938427287));
#8150=CARTESIAN_POINT('Ctrl Pts',(0.225444644405621,-3.24952839182458,7.30988852205161));
#8151=CARTESIAN_POINT('Ctrl Pts',(0.1086266700814,-3.26820558032915,7.42674224413357));
#8152=CARTESIAN_POINT('Ctrl Pts',(-0.0755568103276177,-3.28901857118917,
7.44826275819282));
#8153=CARTESIAN_POINT('Ctrl Pts',(-0.210876101071928,-3.30779418668607,
7.34037569434887));
#8154=CARTESIAN_POINT('Ctrl Pts',(-0.242158837615405,-3.32449655055692,
7.19981012826506));
#8155=CARTESIAN_POINT('Ctrl Pts',(-0.218482747686626,-3.33702480679517,
7.09510428287159));
#8156=CARTESIAN_POINT('Ctrl Pts',(-0.151258418917599,-3.349549304472,7.01092210100317));
#8157=CARTESIAN_POINT('Ctrl Pts',(-0.0544388795806348,-3.36206501623859,
6.96426376579124));
#8158=CARTESIAN_POINT('Ctrl Pts',(0.0529848938244735,-3.37456676113353,
6.96431686779002));
#8159=CARTESIAN_POINT('Ctrl Pts',(0.149618681042139,-3.38704954076379,7.0108168542326));
#8160=CARTESIAN_POINT('Ctrl Pts',(0.216294125348177,-3.39950831444022,7.09454634215613));
#8161=CARTESIAN_POINT('Ctrl Pts',(0.240082283609214,-3.41193813883908,7.19864862883354));
#8162=CARTESIAN_POINT('Ctrl Pts',(0.216301417199454,-3.42433422652378,7.30245308275509));
#8163=CARTESIAN_POINT('Ctrl Pts',(0.155624789134382,-3.43566184662336,7.37854450982395));
#8164=CARTESIAN_POINT('Ctrl Pts',(0.0792338751048572,-3.44592835125056,
7.42061757097289));
#8165=CARTESIAN_POINT('Ctrl Pts',(-0.0236947435290427,-3.45821303575049,
7.43830643547426));
#8166=CARTESIAN_POINT('Ctrl Pts',(-0.1515457831225,-3.47349927012097,7.39355105926792));
#8167=CARTESIAN_POINT('Ctrl Pts',(-0.237353326682969,-3.49171555422899,
7.25657816758057));
#8168=CARTESIAN_POINT('Ctrl Pts',(-0.219180338240666,-3.50979141387795,
7.09733539274298));
#8169=CARTESIAN_POINT('Ctrl Pts',(-0.106639336531097,-3.52771395650611,
6.98511360449985));
#8170=CARTESIAN_POINT('Ctrl Pts',(0.049865171992709,-3.54547134962642,6.96768469168436));
#8171=CARTESIAN_POINT('Ctrl Pts',(0.181721726166896,-3.56305313157731,7.05095143559938));
#8172=CARTESIAN_POINT('Ctrl Pts',(0.215498137389901,-3.57464974765708,7.14788703905096));
#8173=CARTESIAN_POINT('Ctrl Pts',(0.215504679516594,-3.58042060914303,7.19637754768492));
#8174=CARTESIAN_POINT('Ctrl Pts',(0.185107472272675,-2.68073719173477,7.19633995373285));
#8175=CARTESIAN_POINT('Ctrl Pts',(0.185101850763769,-2.68569596220842,7.23800674867565));
#8176=CARTESIAN_POINT('Ctrl Pts',(0.156058199319024,-2.69556022858565,7.32034333803071));
#8177=CARTESIAN_POINT('Ctrl Pts',(0.0462369377041908,-2.71016597633029,
7.38909331331611));
#8178=CARTESIAN_POINT('Ctrl Pts',(-0.0808600379235311,-2.72459415027127,
7.37446486049346));
#8179=CARTESIAN_POINT('Ctrl Pts',(-0.170106237630621,-2.73885403619876,
7.28488979381794));
#8180=CARTESIAN_POINT('Ctrl Pts',(-0.183880616709954,-2.75295769295724,
7.16056856294843));
#8181=CARTESIAN_POINT('Ctrl Pts',(-0.117863262566178,-2.76691743614216,
7.05587052443364));
#8182=CARTESIAN_POINT('Ctrl Pts',(-0.0020314316850335,-2.7807468107492,
7.01551272108977));
#8183=CARTESIAN_POINT('Ctrl Pts',(0.10837582499231,-2.79395216768506,7.05438162297723));
#8184=CARTESIAN_POINT('Ctrl Pts',(0.170462788399269,-2.80656117379754,7.14577794914887));
#8185=CARTESIAN_POINT('Ctrl Pts',(0.170483716515046,-2.818596730844,7.25120669361347));
#8186=CARTESIAN_POINT('Ctrl Pts',(0.11623013408604,-2.82957663370843,7.33066673575509));
#8187=CARTESIAN_POINT('Ctrl Pts',(0.0391429351448043,-2.83952479252818,
7.36762207289601));
#8188=CARTESIAN_POINT('Ctrl Pts',(-0.0375831622377559,-2.84845722206348,
7.36766609159734));
#8189=CARTESIAN_POINT('Ctrl Pts',(-0.106590866905911,-2.85737386804714,
7.33437242450682));
#8190=CARTESIAN_POINT('Ctrl Pts',(-0.154323772729316,-2.86627970238647,
7.27455761393419));
#8191=CARTESIAN_POINT('Ctrl Pts',(-0.171301646699268,-2.87517996511473,
7.20003709996095));
#8192=CARTESIAN_POINT('Ctrl Pts',(-0.154317119566702,-2.88407962497398,
7.1253713308374));
#8193=CARTESIAN_POINT('Ctrl Pts',(-0.106586603192965,-2.89298402606097,
7.06580203076649));
#8194=CARTESIAN_POINT('Ctrl Pts',(-0.0146581859250508,-2.9048694987715,
7.02086680405053));
#8195=CARTESIAN_POINT('Ctrl Pts',(0.119679747928827,-2.91976334307369,7.05112432742094));
#8196=CARTESIAN_POINT('Ctrl Pts',(0.192359619789719,-2.9377356556885,7.20129666148723));
#8197=CARTESIAN_POINT('Ctrl Pts',(0.119710574570271,-2.95584663711404,7.35261634156035));
#8198=CARTESIAN_POINT('Ctrl Pts',(-0.0454133776145315,-2.97413387650899,
7.39082897056735));
#8199=CARTESIAN_POINT('Ctrl Pts',(-0.179953115079168,-2.99263280954147,
7.28410167764536));
#8200=CARTESIAN_POINT('Ctrl Pts',(-0.180187116386609,-3.00981476342207,
7.12511842248155));
#8201=CARTESIAN_POINT('Ctrl Pts',(-0.080455868059763,-3.02563503905427,
7.02585734601489));
#8202=CARTESIAN_POINT('Ctrl Pts',(0.0461874797537591,-3.04003938796267,
7.01117283714634));
#8203=CARTESIAN_POINT('Ctrl Pts',(0.155889163671215,-3.05462162210191,7.07988905593192));
#8204=CARTESIAN_POINT('Ctrl Pts',(0.192002101108853,-3.06692816231653,7.18278090837932));
#8205=CARTESIAN_POINT('Ctrl Pts',(0.177695431363444,-3.07687134320315,7.26607724746195));
#8206=CARTESIAN_POINT('Ctrl Pts',(0.136780671630806,-3.08688063865225,7.34064380608613));
#8207=CARTESIAN_POINT('Ctrl Pts',(0.0421316192783748,-3.0995177452559,7.40052761266016));
#8208=CARTESIAN_POINT('Ctrl Pts',(-0.0934338623745871,-3.11489020621722,
7.38555268889591));
#8209=CARTESIAN_POINT('Ctrl Pts',(-0.191368949641329,-3.13047459530452,
7.28805591492407));
#8210=CARTESIAN_POINT('Ctrl Pts',(-0.207391636243208,-3.1462741944362,7.14884163693624));
#8211=CARTESIAN_POINT('Ctrl Pts',(-0.132098549251811,-3.16229064327564,
7.02839785341959));
#8212=CARTESIAN_POINT('Ctrl Pts',(0.00369007158893442,-3.17852431513169,
6.98052015501029));
#8213=CARTESIAN_POINT('Ctrl Pts',(0.14147140548659,-3.19497417066394,7.02842015914195));
#8214=CARTESIAN_POINT('Ctrl Pts',(0.220404755355712,-3.21163773974047,7.1533143737985));
#8215=CARTESIAN_POINT('Ctrl Pts',(0.204040148119795,-3.22851185815579,7.30213076349379));
#8216=CARTESIAN_POINT('Ctrl Pts',(0.0973630617653471,-3.24559011238179,
7.40912719498989));
#8217=CARTESIAN_POINT('Ctrl Pts',(-0.0724753624674162,-3.26478678833049,
7.42926923462765));
#8218=CARTESIAN_POINT('Ctrl Pts',(-0.198857150771922,-3.28228664005936,
7.32901755401093));
#8219=CARTESIAN_POINT('Ctrl Pts',(-0.228415618223813,-3.29800120150021,
7.19676443740428));
#8220=CARTESIAN_POINT('Ctrl Pts',(-0.206056653052093,-3.30986343736228,
7.09761156829177));
#8221=CARTESIAN_POINT('Ctrl Pts',(-0.142055048123301,-3.32179879095291,
7.01733731331786));
#8222=CARTESIAN_POINT('Ctrl Pts',(-0.0492154972805245,-3.33380382681927,
6.9725138159443));
#8223=CARTESIAN_POINT('Ctrl Pts',(0.0545114782345651,-3.34587484328919,
6.97248829472171));
#8224=CARTESIAN_POINT('Ctrl Pts',(0.148474547415015,-3.35800808352178,7.01761622718362));
#8225=CARTESIAN_POINT('Ctrl Pts',(0.213783582718699,-3.37019943651325,7.09950448341927));
#8226=CARTESIAN_POINT('Ctrl Pts',(0.237296599865736,-3.38244484532487,7.20204554953723));
#8227=CARTESIAN_POINT('Ctrl Pts',(0.213786034721385,-3.39473983718185,7.30502757685629));
#8228=CARTESIAN_POINT('Ctrl Pts',(0.153251203560767,-3.40605176457476,7.38106061938234));
#8229=CARTESIAN_POINT('Ctrl Pts',(0.0765239927439651,-3.41636484949048,
7.42336069496949));
#8230=CARTESIAN_POINT('Ctrl Pts',(-0.0273847389731562,-3.42876839128249,
7.44126747332444));
#8231=CARTESIAN_POINT('Ctrl Pts',(-0.157533033535677,-3.44431985844659,
7.3959554283747));
#8232=CARTESIAN_POINT('Ctrl Pts',(-0.245963473728323,-3.46304035049211,
7.25534056816814));
#8233=CARTESIAN_POINT('Ctrl Pts',(-0.227377089922609,-3.48180333014707,
7.09001457354066));
#8234=CARTESIAN_POINT('Ctrl Pts',(-0.10959705092368,-3.50059017332273,6.9721779507632));
#8235=CARTESIAN_POINT('Ctrl Pts',(0.0560250788067464,-3.51938704187467,
6.95348154924594));
#8236=CARTESIAN_POINT('Ctrl Pts',(0.197052436429245,-3.53816884599807,7.04220437160198));
#8237=CARTESIAN_POINT('Ctrl Pts',(0.233628963287126,-3.55068088369041,7.14674488416437));
#8238=CARTESIAN_POINT('Ctrl Pts',(0.233636036508055,-3.55692022758386,7.19917188482486));
#8239=CARTESIAN_POINT('Ctrl Pts',(0.214878329241221,-2.68071167631188,7.19634700688545));
#8240=CARTESIAN_POINT('Ctrl Pts',(0.21487182329556,-2.68645061434203,7.24456927394994));
#8241=CARTESIAN_POINT('Ctrl Pts',(0.181215095804958,-2.69789401566424,7.34010917676144));
#8242=CARTESIAN_POINT('Ctrl Pts',(0.0537659785169842,-2.71484126590492,
7.41988663023413));
#8243=CARTESIAN_POINT('Ctrl Pts',(-0.09373371851528,-2.73158585390756,7.40290940748877));
#8244=CARTESIAN_POINT('Ctrl Pts',(-0.197166167452985,-2.74811534933935,
7.29903046327851));
#8245=CARTESIAN_POINT('Ctrl Pts',(-0.213034321110582,-2.76443051525134,
7.15519994000744));
#8246=CARTESIAN_POINT('Ctrl Pts',(-0.136819975557523,-2.78052820707376,
7.03450142161169));
#8247=CARTESIAN_POINT('Ctrl Pts',(-0.00375351882357425,-2.79640902509429,
6.98826242279056));
#8248=CARTESIAN_POINT('Ctrl Pts',(0.122333193616463,-2.81149365697418,7.03278955833157));
#8249=CARTESIAN_POINT('Ctrl Pts',(0.192744669714971,-2.82581172202087,7.13664478499631));
#8250=CARTESIAN_POINT('Ctrl Pts',(0.192647881053207,-2.8393914952052,7.25560741643829));
#8251=CARTESIAN_POINT('Ctrl Pts',(0.131770645966198,-2.85169082997991,7.34455022261805));
#8252=CARTESIAN_POINT('Ctrl Pts',(0.0459939732724772,-2.86275697963967,
7.3855948352218));
#8253=CARTESIAN_POINT('Ctrl Pts',(-0.0388130362826423,-2.87262995943921,
7.38558203095042));
#8254=CARTESIAN_POINT('Ctrl Pts',(-0.114539127899638,-2.88241859001702,
7.34897184256002));
#8255=CARTESIAN_POINT('Ctrl Pts',(-0.166511534095061,-2.89212570551886,
7.28373270044754));
#8256=CARTESIAN_POINT('Ctrl Pts',(-0.184810079874889,-2.90175391362293,
7.20310188788887));
#8257=CARTESIAN_POINT('Ctrl Pts',(-0.166499070669721,-2.91130664969882,
7.12297856836614));
#8258=CARTESIAN_POINT('Ctrl Pts',(-0.115640722633783,-2.92078670707761,
7.05960552710051));
#8259=CARTESIAN_POINT('Ctrl Pts',(-0.0185035951711087,-2.93333502747441,
7.01225906285182));
#8260=CARTESIAN_POINT('Ctrl Pts',(0.121384202754409,-2.94885754279125,7.04432810744503));
#8261=CARTESIAN_POINT('Ctrl Pts',(0.195134680693374,-2.96725491613172,7.19836545333501));
#8262=CARTESIAN_POINT('Ctrl Pts',(0.121492212412953,-2.98545720090378,7.35011748851036));
#8263=CARTESIAN_POINT('Ctrl Pts',(-0.0415756095516308,-3.00350071291157,
7.38713785532324));
#8264=CARTESIAN_POINT('Ctrl Pts',(-0.171471644948999,-3.02142390268615,
7.28320999930232));
#8265=CARTESIAN_POINT('Ctrl Pts',(-0.171122013040012,-3.03777918677307,
7.1319049638478));
#8266=CARTESIAN_POINT('Ctrl Pts',(-0.0773985344224403,-3.05261903400135,
7.039049711749));
#8267=CARTESIAN_POINT('Ctrl Pts',(0.0399833773515873,-3.06597019341009,
7.02566105807932));
#8268=CARTESIAN_POINT('Ctrl Pts',(0.140369924424537,-3.07933150614831,7.08880680890486));
#8269=CARTESIAN_POINT('Ctrl Pts',(0.172952186649219,-3.09049185762763,7.18213910205967));
#8270=CARTESIAN_POINT('Ctrl Pts',(0.160047639831177,-3.09944207648492,7.2570980192185));
#8271=CARTESIAN_POINT('Ctrl Pts',(0.123360578173005,-3.10841052070708,7.32389555825651));
#8272=CARTESIAN_POINT('Ctrl Pts',(0.0390364069690545,-3.11966187978331,
7.37708457574868));
#8273=CARTESIAN_POINT('Ctrl Pts',(-0.0806839027680721,-3.13324221912812,
7.36370840776829));
#8274=CARTESIAN_POINT('Ctrl Pts',(-0.166516225814016,-3.14691808423354,
7.27808190977155));
#8275=CARTESIAN_POINT('Ctrl Pts',(-0.1803885024237,-3.16070433204962,7.15662107539426));
#8276=CARTESIAN_POINT('Ctrl Pts',(-0.114933495650407,-3.17461568751952,
7.05207571305458));
#8277=CARTESIAN_POINT('Ctrl Pts',(0.00258664962602312,-3.18866585403527,
7.01070631425415));
#8278=CARTESIAN_POINT('Ctrl Pts',(0.121500437060258,-3.20286770222029,7.05209149218014));
#8279=CARTESIAN_POINT('Ctrl Pts',(0.189515967342179,-3.21723327862761,7.15974852768408));
#8280=CARTESIAN_POINT('Ctrl Pts',(0.175418084641306,-3.2317720828774,7.2879569750776));
#8281=CARTESIAN_POINT('Ctrl Pts',(0.0834767702888784,-3.24649681310668,
7.38019750575045));
#8282=CARTESIAN_POINT('Ctrl Pts',(-0.063118475428651,-3.26307103030429,
7.39764002158794));
#8283=CARTESIAN_POINT('Ctrl Pts',(-0.172586769126297,-3.27822107611759,
7.31094414714426));
#8284=CARTESIAN_POINT('Ctrl Pts',(-0.198306357495174,-3.29187213671086,
7.19607145757355));
#8285=CARTESIAN_POINT('Ctrl Pts',(-0.178855476148038,-3.30220421737521,
7.10971022421916));
#8286=CARTESIAN_POINT('Ctrl Pts',(-0.122973787180029,-3.31263115861789,
7.03956593295181));
#8287=CARTESIAN_POINT('Ctrl Pts',(-0.041619423464239,-3.32315369917206,
7.00024936303785));
#8288=CARTESIAN_POINT('Ctrl Pts',(0.0496224608427707,-3.33377249093432,
7.0001876752484));
#8289=CARTESIAN_POINT('Ctrl Pts',(0.132615977620369,-3.34448764766654,7.04000114288187));
#8290=CARTESIAN_POINT('Ctrl Pts',(0.190567079631117,-3.35529935310258,7.11259019946977));
#8291=CARTESIAN_POINT('Ctrl Pts',(0.211557095963147,-3.36620709548451,7.20391423560445));
#8292=CARTESIAN_POINT('Ctrl Pts',(0.19056766958691,-3.3772106311537,7.29608667824698));
#8293=CARTESIAN_POINT('Ctrl Pts',(0.136166978738086,-3.38738386597841,7.36449481817329));
#8294=CARTESIAN_POINT('Ctrl Pts',(0.0668637166489791,-3.39670087321399,
7.40273214763341));
#8295=CARTESIAN_POINT('Ctrl Pts',(-0.0273632555059043,-3.40795054895204,
7.41900543577496));
#8296=CARTESIAN_POINT('Ctrl Pts',(-0.146177376821207,-3.42214234210721,
7.37782632931633));
#8297=CARTESIAN_POINT('Ctrl Pts',(-0.227756280424957,-3.43937189049888,
7.24854197729575));
#8298=CARTESIAN_POINT('Ctrl Pts',(-0.210735924661904,-3.45679498612433,
7.09500736118589));
#8299=CARTESIAN_POINT('Ctrl Pts',(-0.100539622313171,-3.4744007837155,6.98440854237947));
#8300=CARTESIAN_POINT('Ctrl Pts',(0.0561077229205953,-3.49218430227486,
6.96647422873777));
#8301=CARTESIAN_POINT('Ctrl Pts',(0.190963235128123,-3.51012426777635,7.05099318661589));
#8302=CARTESIAN_POINT('Ctrl Pts',(0.226408417556183,-3.5221978574293,7.15180919947803));
#8303=CARTESIAN_POINT('Ctrl Pts',(0.226415268139349,-3.52824081079723,7.20258599999129));
#8304=CARTESIAN_POINT('Ctrl Pts',(0.233538303779023,-2.65759637264774,7.19910047958883));
#8305=CARTESIAN_POINT('Ctrl Pts',(0.23353123930546,-2.66382799186311,7.25146257244798));
#8306=CARTESIAN_POINT('Ctrl Pts',(0.19696745884569,-2.6763073269123,7.3556708689899));
#8307=CARTESIAN_POINT('Ctrl Pts',(0.0569730084398323,-2.69494130883234,
7.44356718383999));
#8308=CARTESIAN_POINT('Ctrl Pts',(-0.106524442685284,-2.71350166413368,
7.42496929134948));
#8309=CARTESIAN_POINT('Ctrl Pts',(-0.222163571737669,-2.73196121008211,
7.3091230299507));
#8310=CARTESIAN_POINT('Ctrl Pts',(-0.240199522465172,-2.75030982448797,
7.14741578501388));
#8311=CARTESIAN_POINT('Ctrl Pts',(-0.154095608050911,-2.76853080499078,
7.01072914726199));
#8312=CARTESIAN_POINT('Ctrl Pts',(-0.00267460687807611,-2.78661147066547,
6.95794871950724));
#8313=CARTESIAN_POINT('Ctrl Pts',(0.14164030899789,-2.8038747511127,7.00878148038353));
#8314=CARTESIAN_POINT('Ctrl Pts',(0.222615117792197,-2.82032946000645,7.12807539253736));
#8315=CARTESIAN_POINT('Ctrl Pts',(0.222566032265283,-2.83598692966601,7.26523101242083));
#8316=CARTESIAN_POINT('Ctrl Pts',(0.152222724280741,-2.85020730425676,7.36808448669668));
#8317=CARTESIAN_POINT('Ctrl Pts',(0.052883269474769,-2.86302436513278,7.41563755649051));
#8318=CARTESIAN_POINT('Ctrl Pts',(-0.0454508997787033,-2.87447229970568,
7.41563379936155));
#8319=CARTESIAN_POINT('Ctrl Pts',(-0.133324971812771,-2.88583102579193,
7.37315841026056));
#8320=CARTESIAN_POINT('Ctrl Pts',(-0.193653504241113,-2.89709830105743,
7.29743342327476));
#8321=CARTESIAN_POINT('Ctrl Pts',(-0.214889368558948,-2.90827301861113,
7.20385133456187));
#8322=CARTESIAN_POINT('Ctrl Pts',(-0.193640662373467,-2.91935338080873,
7.11091006412822));
#8323=CARTESIAN_POINT('Ctrl Pts',(-0.134699243008982,-2.93033890052561,
7.03748141089585));
#8324=CARTESIAN_POINT('Ctrl Pts',(-0.0222774827983604,-2.94485821758379,
6.98270915909811));
#8325=CARTESIAN_POINT('Ctrl Pts',(0.139091593640502,-2.96276591757136,7.01987612520336));
#8326=CARTESIAN_POINT('Ctrl Pts',(0.223437037797074,-2.98386877798849,7.196730445542));
#8327=CARTESIAN_POINT('Ctrl Pts',(0.139257378147977,-3.00458867914989,7.36934332497687));
#8328=CARTESIAN_POINT('Ctrl Pts',(-0.0447572277219394,-3.02493383754544,
7.41066476064657));
#8329=CARTESIAN_POINT('Ctrl Pts',(-0.189286778967101,-3.04491624179778,
7.29436254156531));
#8330=CARTESIAN_POINT('Ctrl Pts',(-0.188403825735976,-3.06291651894871,
7.12780952218904));
#8331=CARTESIAN_POINT('Ctrl Pts',(-0.0863353928960517,-3.07904135259068,
7.02711014487625));
#8332=CARTESIAN_POINT('Ctrl Pts',(0.0398108006740648,-3.09337910804554,
7.01296405421245));
#8333=CARTESIAN_POINT('Ctrl Pts',(0.146208508440029,-3.10755812551401,7.08021718201157));
#8334=CARTESIAN_POINT('Ctrl Pts',(0.180131861009168,-3.11924556686056,7.17807435840992));
#8335=CARTESIAN_POINT('Ctrl Pts',(0.16670128029989,-3.12852929709267,7.25582324597245));
#8336=CARTESIAN_POINT('Ctrl Pts',(0.128849181526771,-3.1377695627669,7.32464682833912));
#8337=CARTESIAN_POINT('Ctrl Pts',(0.0427116800450749,-3.149239893477,7.37870702037907));
#8338=CARTESIAN_POINT('Ctrl Pts',(-0.0777006583769931,-3.16289693813138,
7.36496356140122));
#8339=CARTESIAN_POINT('Ctrl Pts',(-0.162663216489806,-3.17646003764126,
7.27980557815832));
#8340=CARTESIAN_POINT('Ctrl Pts',(-0.175962341940663,-3.18994594112167,
7.16090735254292));
#8341=CARTESIAN_POINT('Ctrl Pts',(-0.112537351249249,-3.20337070954953,
7.0601179958768));
#8342=CARTESIAN_POINT('Ctrl Pts',(-0.000481216033886487,-3.21675127677844,
7.02095151118088));
#8343=CARTESIAN_POINT('Ctrl Pts',(0.111296697656111,-3.23010475115374,7.06011758513708));
#8344=CARTESIAN_POINT('Ctrl Pts',(0.174298843579563,-3.24344811181235,7.16029176874159));
#8345=CARTESIAN_POINT('Ctrl Pts',(0.161127262848427,-3.25680162593276,7.27804919975625));
#8346=CARTESIAN_POINT('Ctrl Pts',(0.0774244337848529,-3.27017623909351,
7.36174389935327));
#8347=CARTESIAN_POINT('Ctrl Pts',(-0.0545258475331624,-3.28508517972487,
7.3771987766231));
#8348=CARTESIAN_POINT('Ctrl Pts',(-0.151842439762883,-3.2985726274777,7.29977278923544));
#8349=CARTESIAN_POINT('Ctrl Pts',(-0.174497392547656,-3.31063449086272,
7.19825771524167));
#8350=CARTESIAN_POINT('Ctrl Pts',(-0.157357750943022,-3.31972130199921,
7.12229297679189));
#8351=CARTESIAN_POINT('Ctrl Pts',(-0.108376416413373,-3.32885327484438,
7.06087320694589));
#8352=CARTESIAN_POINT('Ctrl Pts',(-0.0373643947482642,-3.33803498700604,
7.02658711572428));
#8353=CARTESIAN_POINT('Ctrl Pts',(0.0420064034120988,-3.34727056328954,
7.02656190673972));
#8354=CARTESIAN_POINT('Ctrl Pts',(0.113992645451419,-3.35656453452081,7.06112022321622));
#8355=CARTESIAN_POINT('Ctrl Pts',(0.164133070511383,-3.36592049244828,7.12395812004847));
#8356=CARTESIAN_POINT('Ctrl Pts',(0.182252226692838,-3.37534284388788,7.20285791598277));
#8357=CARTESIAN_POINT('Ctrl Pts',(0.164132253563985,-3.3848345376368,7.28237529070212));
#8358=CARTESIAN_POINT('Ctrl Pts',(0.117236828749836,-3.39360290117376,7.34133619710266));
#8359=CARTESIAN_POINT('Ctrl Pts',(0.0575242319280615,-3.40162933393007,
7.37427980345525));
#8360=CARTESIAN_POINT('Ctrl Pts',(-0.0236535488582548,-3.41132057199507,
7.38829815085827));
#8361=CARTESIAN_POINT('Ctrl Pts',(-0.126036636133201,-3.42354719842553,
7.35282484173021));
#8362=CARTESIAN_POINT('Ctrl Pts',(-0.196447507190014,-3.43841077228126,
7.24130556418034));
#8363=CARTESIAN_POINT('Ctrl Pts',(-0.181786690767014,-3.45347315019531,
7.10855232056132));
#8364=CARTESIAN_POINT('Ctrl Pts',(-0.0862766704206619,-3.46874015439278,
7.0125916034523));
#8365=CARTESIAN_POINT('Ctrl Pts',(0.0500732682335706,-3.48421890261266,
6.99687835328418));
#8366=CARTESIAN_POINT('Ctrl Pts',(0.168070534236532,-3.49990825557829,7.07070558821891));
#8367=CARTESIAN_POINT('Ctrl Pts',(0.199310683862651,-3.51051845488447,7.15928045848644));
#8368=CARTESIAN_POINT('Ctrl Pts',(0.199316725929205,-3.5158482093806,7.20406450104937));
#8369=CARTESIAN_POINT('Ctrl Pts',(0.226807069374228,-2.62874525353582,7.20253314673028));
#8370=CARTESIAN_POINT('Ctrl Pts',(0.226800193170563,-2.63481079862087,7.25349977739365));
#8371=CARTESIAN_POINT('Ctrl Pts',(0.191272485389705,-2.64698867836095,7.35528689274925));
#8372=CARTESIAN_POINT('Ctrl Pts',(0.0533110857492899,-2.66537236048706,
7.44226188191812));
#8373=CARTESIAN_POINT('Ctrl Pts',(-0.109667876964825,-2.68386464624667,
7.42398792365078));
#8374=CARTESIAN_POINT('Ctrl Pts',(-0.226294478669585,-2.70244725643931,
7.30754504264378));
#8375=CARTESIAN_POINT('Ctrl Pts',(-0.244914583118051,-2.72110552668272,
7.14309248345841));
#8376=CARTESIAN_POINT('Ctrl Pts',(-0.15668266949549,-2.73982241025182,7.00250636322875));
#8377=CARTESIAN_POINT('Ctrl Pts',(0.000360275167344028,-2.75858136287757,
6.94746740129157));
#8378=CARTESIAN_POINT('Ctrl Pts',(0.151688784472103,-2.77666942058048,7.00049231569798));
#8379=CARTESIAN_POINT('Ctrl Pts',(0.23748865440538,-2.79406856806348,7.12654303181867));
#8380=CARTESIAN_POINT('Ctrl Pts',(0.23761695716689,-2.81076579754878,7.27280866250993));
#8381=CARTESIAN_POINT('Ctrl Pts',(0.162117527595802,-2.82605484913246,7.38348851179891));
#8382=CARTESIAN_POINT('Ctrl Pts',(0.0545882621468924,-2.83993173646103,
7.43504994553777));
#8383=CARTESIAN_POINT('Ctrl Pts',(-0.0524979360585502,-2.85239907298462,
7.43511222101232));
#8384=CARTESIAN_POINT('Ctrl Pts',(-0.148769496310483,-2.86483915988807,
7.38865172607033));
#8385=CARTESIAN_POINT('Ctrl Pts',(-0.215254024761476,-2.87724759240759,
7.30530082688861));
#8386=CARTESIAN_POINT('Ctrl Pts',(-0.238821796662854,-2.88961903583731,
7.20171142411695));
#8387=CARTESIAN_POINT('Ctrl Pts',(-0.215238237798196,-2.90194974810172,
7.09827776484272));
#8388=CARTESIAN_POINT('Ctrl Pts',(-0.149364834601404,-2.91423378360337,
7.01614108176756));
#8389=CARTESIAN_POINT('Ctrl Pts',(-0.0231308706748203,-2.93054559789587,
6.95454388888739));
#8390=CARTESIAN_POINT('Ctrl Pts',(0.159420173978833,-2.95079940372033,6.99624966262056));
#8391=CARTESIAN_POINT('Ctrl Pts',(0.255873437394368,-2.97485199097034,7.19763372613105));
#8392=CARTESIAN_POINT('Ctrl Pts',(0.15957313095635,-2.99862366344323,7.39576846719451));
#8393=CARTESIAN_POINT('Ctrl Pts',(-0.0525587099637037,-3.02208750782865,
7.44363039833475));
#8394=CARTESIAN_POINT('Ctrl Pts',(-0.219931950941677,-3.04522091566892,
7.30913177612171));
#8395=CARTESIAN_POINT('Ctrl Pts',(-0.218965218054516,-3.06610519788919,
7.11593913699533));
#8396=CARTESIAN_POINT('Ctrl Pts',(-0.100501511682712,-3.08482617518605,
6.99907504856024));
#8397=CARTESIAN_POINT('Ctrl Pts',(0.0458164463407195,-3.10146601073649,
6.98269678592085));
#8398=CARTESIAN_POINT('Ctrl Pts',(0.168999497221885,-3.11788828933047,7.06061891332887));
#8399=CARTESIAN_POINT('Ctrl Pts',(0.208122474292555,-3.13139648646481,7.17367059053374));
#8400=CARTESIAN_POINT('Ctrl Pts',(0.192637292346469,-3.14209220126933,7.26321724442717));
#8401=CARTESIAN_POINT('Ctrl Pts',(0.149112713706763,-3.15271566117018,7.34232079626982));
#8402=CARTESIAN_POINT('Ctrl Pts',(0.0503918987656031,-3.16586237028332,
7.40415778281572));
#8403=CARTESIAN_POINT('Ctrl Pts',(-0.0867200805671385,-3.18142249838002,
7.38835737794119));
#8404=CARTESIAN_POINT('Ctrl Pts',(-0.182700211691555,-3.19677179886155,
7.29191823673));
#8405=CARTESIAN_POINT('Ctrl Pts',(-0.197437125539796,-3.21191412401389,
7.1584636059683));
#8406=CARTESIAN_POINT('Ctrl Pts',(-0.126707005483683,-3.22685574481417,
7.04645677722269));
#8407=CARTESIAN_POINT('Ctrl Pts',(-0.00319094454791707,-3.24160375982955,
7.00352504192919));
#8408=CARTESIAN_POINT('Ctrl Pts',(0.11856508268551,-3.25616661068809,7.04643998602982));
#8409=CARTESIAN_POINT('Ctrl Pts',(0.186244643735728,-3.270554152578,7.15453132429662));
#8410=CARTESIAN_POINT('Ctrl Pts',(0.171956140631049,-3.28477480105648,7.27987318903316));
#8411=CARTESIAN_POINT('Ctrl Pts',(0.083770472898142,-3.29884525026963,7.36768722105074));
#8412=CARTESIAN_POINT('Ctrl Pts',(-0.0531987671053138,-3.31432198686421,
7.3833677722724));
#8413=CARTESIAN_POINT('Ctrl Pts',(-0.152299260177419,-3.32810268380143,
7.3039248465455));
#8414=CARTESIAN_POINT('Ctrl Pts',(-0.174981847078137,-3.34025604687833,
7.20166189370968));
#8415=CARTESIAN_POINT('Ctrl Pts',(-0.157808289885975,-3.34932803257825,
7.12584849313869));
#8416=CARTESIAN_POINT('Ctrl Pts',(-0.109299772760072,-3.35836163086098,
7.06515673754344));
#8417=CARTESIAN_POINT('Ctrl Pts',(-0.0396742128789388,-3.36736140818118,
7.03162683559205));
#8418=CARTESIAN_POINT('Ctrl Pts',(0.0374060865469686,-3.37633248399835,
7.03167814263163));
#8419=CARTESIAN_POINT('Ctrl Pts',(0.106662131123058,-3.38527943925005,7.06501065247445));
#8420=CARTESIAN_POINT('Ctrl Pts',(0.154443458609935,-3.39420766474773,7.12500716832091));
#8421=CARTESIAN_POINT('Ctrl Pts',(0.171513122490573,-3.40312176328236,7.19966018133591));
#8422=CARTESIAN_POINT('Ctrl Pts',(0.154448810128273,-3.4120273277969,7.27423689345863));
#8423=CARTESIAN_POINT('Ctrl Pts',(0.110761145556717,-3.42018708551772,7.32906401524711));
#8424=CARTESIAN_POINT('Ctrl Pts',(0.0555624170066066,-3.42760636575424,
7.35948454642012));
#8425=CARTESIAN_POINT('Ctrl Pts',(-0.0190556043401421,-3.43651328476221,
7.37233115593073));
#8426=CARTESIAN_POINT('Ctrl Pts',(-0.112331457345363,-3.44766009018625,
7.33983175331251));
#8427=CARTESIAN_POINT('Ctrl Pts',(-0.175704040546785,-3.46107387540665,
7.23909310909943));
#8428=CARTESIAN_POINT('Ctrl Pts',(-0.162425909441732,-3.47454209114925,
7.12040978273045));
#8429=CARTESIAN_POINT('Ctrl Pts',(-0.0776194368412568,-3.48808204867214,
7.03542354959143));
#8430=CARTESIAN_POINT('Ctrl Pts',(0.0424348764358349,-3.50170807079122,
7.02170483465243));
#8431=CARTESIAN_POINT('Ctrl Pts',(0.145618410675924,-3.51543992220036,7.08642673131801));
#8432=CARTESIAN_POINT('Ctrl Pts',(0.172745123919546,-3.52466866031849,7.16348700295488));
#8433=CARTESIAN_POINT('Ctrl Pts',(0.172750382832977,-3.5293075892768,7.20246628278216));
#8434=CARTESIAN_POINT('Ctrl Pts',(0.208975500613569,-2.62021022067982,7.20354649629684));
#8435=CARTESIAN_POINT('Ctrl Pts',(0.208969152515337,-2.62580992044147,7.25059879342368));
#8436=CARTESIAN_POINT('Ctrl Pts',(0.176200542181115,-2.63705663059552,7.34462698401245));
#8437=CARTESIAN_POINT('Ctrl Pts',(0.0482380022249738,-2.65411768985976,
7.42545084377329));
#8438=CARTESIAN_POINT('Ctrl Pts',(-0.103720983462279,-2.67135555018703,
7.40853032917249));
#8439=CARTESIAN_POINT('Ctrl Pts',(-0.213091232946899,-2.68876552670636,
7.29953341464567));
#8440=CARTESIAN_POINT('Ctrl Pts',(-0.230778210290289,-2.70633773804461,
7.14465406518129));
#8441=CARTESIAN_POINT('Ctrl Pts',(-0.147346836969467,-2.7240630897452,7.01142232753577));
#8442=CARTESIAN_POINT('Ctrl Pts',(0.00219669286606783,-2.74193073856756,
6.95883670315601));
#8443=CARTESIAN_POINT('Ctrl Pts',(0.147274876105101,-2.75926262337493,7.00950168746689));
#8444=CARTESIAN_POINT('Ctrl Pts',(0.230088843486711,-2.77603178187632,7.13094085128893));
#8445=CARTESIAN_POINT('Ctrl Pts',(0.230334378766964,-2.7922170622316,7.2727313032445));
#8446=CARTESIAN_POINT('Ctrl Pts',(0.156818756385348,-2.80712034812938,7.3807101094845));
#8447=CARTESIAN_POINT('Ctrl Pts',(0.0514599371458473,-2.82071832270221,
7.4312969017612));
#8448=CARTESIAN_POINT('Ctrl Pts',(-0.053949273106916,-2.83298814079633,
7.43141235157773));
#8449=CARTESIAN_POINT('Ctrl Pts',(-0.149162803673346,-2.84528639082816,
7.38552243933886));
#8450=CARTESIAN_POINT('Ctrl Pts',(-0.215239756886203,-2.85760759853358,
7.30277372032405));
#8451=CARTESIAN_POINT('Ctrl Pts',(-0.238803777980285,-2.8699484285224,7.19943437440153));
#8452=CARTESIAN_POINT('Ctrl Pts',(-0.215229520115252,-2.88230106367663,
7.09576020758005));
#8453=CARTESIAN_POINT('Ctrl Pts',(-0.148939420593191,-2.89466611719909,
7.01303450291724));
#8454=CARTESIAN_POINT('Ctrl Pts',(-0.0213325673406164,-2.91115883006794,
6.95066970086975));
#8455=CARTESIAN_POINT('Ctrl Pts',(0.164620027801451,-2.93177219578512,6.99277194403154));
#8456=CARTESIAN_POINT('Ctrl Pts',(0.264140345441926,-2.95647425946544,7.1994621312341));
#8457=CARTESIAN_POINT('Ctrl Pts',(0.164728852326112,-2.98110257359385,7.4050323399217));
#8458=CARTESIAN_POINT('Ctrl Pts',(-0.0569443318317078,-3.0056223317769,
7.45549377665849));
#8459=CARTESIAN_POINT('Ctrl Pts',(-0.233655234082383,-3.02999749647669,
7.31403792989835));
#8460=CARTESIAN_POINT('Ctrl Pts',(-0.232974963582391,-3.05218001599301,
7.10874779894472));
#8461=CARTESIAN_POINT('Ctrl Pts',(-0.106388781594654,-3.07219040709644,
6.98361852003422));
#8462=CARTESIAN_POINT('Ctrl Pts',(0.0509166303138672,-3.09006797134932,
6.96587840747777));
#8463=CARTESIAN_POINT('Ctrl Pts',(0.184107855620212,-3.10781070899736,7.049980356836));
#8464=CARTESIAN_POINT('Ctrl Pts',(0.22667112837476,-3.12246458039756,7.17268484719045));
#8465=CARTESIAN_POINT('Ctrl Pts',(0.209820378030098,-3.13411078817146,7.27022208122515));
#8466=CARTESIAN_POINT('Ctrl Pts',(0.162337133022933,-3.14570167635411,7.35655665500323));
#8467=CARTESIAN_POINT('Ctrl Pts',(0.0543381183921439,-3.16007989039251,
7.42429494476246));
#8468=CARTESIAN_POINT('Ctrl Pts',(-0.0962325781952025,-3.17715803206852,
7.40702433836543));
#8469=CARTESIAN_POINT('Ctrl Pts',(-0.201968741853417,-3.19405130244851,
7.30086969204493));
#8470=CARTESIAN_POINT('Ctrl Pts',(-0.218281002748809,-3.21075559415295,
7.15358183271638));
#8471=CARTESIAN_POINT('Ctrl Pts',(-0.140111375872412,-3.22726635027305,
7.02973402788688));
#8472=CARTESIAN_POINT('Ctrl Pts',(-0.0034165106286539,-3.24358092971903,
6.98220471253357));
#8473=CARTESIAN_POINT('Ctrl Pts',(0.131391629234701,-3.25969776110748,7.02971930828623));
#8474=CARTESIAN_POINT('Ctrl Pts',(0.206292361264499,-3.27561627696566,7.14937558433617));
#8475=CARTESIAN_POINT('Ctrl Pts',(0.190461110925075,-3.29133937308174,7.2879807743595));
#8476=CARTESIAN_POINT('Ctrl Pts',(0.0930770533573671,-3.30686565126976,
7.38489251842631));
#8477=CARTESIAN_POINT('Ctrl Pts',(-0.0577831284559989,-3.32390509058752,
7.40207685645854));
#8478=CARTESIAN_POINT('Ctrl Pts',(-0.166431009430519,-3.33902296977876,
7.31480305950528));
#8479=CARTESIAN_POINT('Ctrl Pts',(-0.191165405660558,-3.35230195988059,
7.20305195896223));
#8480=CARTESIAN_POINT('Ctrl Pts',(-0.172430795699987,-3.36218424465458,
7.12046761230825));
#8481=CARTESIAN_POINT('Ctrl Pts',(-0.119735198215102,-3.37199121037803,
7.05459706635593));
#8482=CARTESIAN_POINT('Ctrl Pts',(-0.0444046399914078,-3.3817262001077,
7.01836103206837));
#8483=CARTESIAN_POINT('Ctrl Pts',(0.0386419326090535,-3.39139119363884,
7.0184564545768));
#8484=CARTESIAN_POINT('Ctrl Pts',(0.1129237126287,-3.40098989064185,7.05425452293928));
#8485=CARTESIAN_POINT('Ctrl Pts',(0.163917462051814,-3.41052478524528,7.11835470673475));
#8486=CARTESIAN_POINT('Ctrl Pts',(0.182015951489857,-3.41999969889282,7.19771033519379));
#8487=CARTESIAN_POINT('Ctrl Pts',(0.163925204547397,-3.42941792680988,7.27656408688283));
#8488=CARTESIAN_POINT('Ctrl Pts',(0.117932620661441,-3.43800234053243,7.33421196773936));
#8489=CARTESIAN_POINT('Ctrl Pts',(0.0601344625788096,-3.44577115500963,
7.36603928463948));
#8490=CARTESIAN_POINT('Ctrl Pts',(-0.017670556131189,-3.45505825853875,
7.3794035026531));
#8491=CARTESIAN_POINT('Ctrl Pts',(-0.114246172587839,-3.46660968997134,
7.34559229118226));
#8492=CARTESIAN_POINT('Ctrl Pts',(-0.179147820429239,-3.48038656567466,
7.2420523320965));
#8493=CARTESIAN_POINT('Ctrl Pts',(-0.165439388560693,-3.4940951352783,7.1213117854776));
#8494=CARTESIAN_POINT('Ctrl Pts',(-0.0797949579373658,-3.50775053636266,
7.03576635961576));
#8495=CARTESIAN_POINT('Ctrl Pts',(0.0401637289317659,-3.52136611451607,
7.02224445826465));
#8496=CARTESIAN_POINT('Ctrl Pts',(0.142198917848681,-3.53496290502824,7.08647253741509));
#8497=CARTESIAN_POINT('Ctrl Pts',(0.168714822472972,-3.54401637293365,7.16206440300629));
#8498=CARTESIAN_POINT('Ctrl Pts',(0.16871996439457,-3.54855210247603,7.20017653463026));
#8499=CARTESIAN_POINT('Ctrl Pts',(0.199999521685004,-2.62021022067982,7.20354528529548));
#8500=CARTESIAN_POINT('Ctrl Pts',(0.19999343949118,-2.6255753643916,7.24862669087077));
#8501=CARTESIAN_POINT('Ctrl Pts',(0.168615691452697,-2.63634781999191,7.33868016798294));
#8502=CARTESIAN_POINT('Ctrl Pts',(0.0459616996448183,-2.65270477799173,
7.41618164971903));
#8503=CARTESIAN_POINT('Ctrl Pts',(-0.0998469869656992,-2.66924595959392,
7.39996507729611));
#8504=CARTESIAN_POINT('Ctrl Pts',(-0.204936181985623,-2.68597304189578,
7.29527847685269));
#8505=CARTESIAN_POINT('Ctrl Pts',(-0.221986969755699,-2.7028797483455,7.14628505326925));
#8506=CARTESIAN_POINT('Ctrl Pts',(-0.141631327334848,-2.71996166380803,
7.01788664502262));
#8507=CARTESIAN_POINT('Ctrl Pts',(0.00270481241442624,-2.73721192504324,
6.96708134679183));
#8508=CARTESIAN_POINT('Ctrl Pts',(0.143039113459417,-2.75397833948373,7.01603761180454));
#8509=CARTESIAN_POINT('Ctrl Pts',(0.223330027417085,-2.77023316539608,7.13370506584288));
#8510=CARTESIAN_POINT('Ctrl Pts',(0.223609433092684,-2.7859516486779,7.2713911725354));
#8511=CARTESIAN_POINT('Ctrl Pts',(0.152101468687107,-2.80045790761646,7.37648984952004));
#8512=CARTESIAN_POINT('Ctrl Pts',(0.0493840180807327,-2.81371750007274,
7.42583309513969));
#8513=CARTESIAN_POINT('Ctrl Pts',(-0.0535656424988984,-2.82570326133932,
7.42596307871198));
#8514=CARTESIAN_POINT('Ctrl Pts',(-0.146731811694293,-2.83773755003964,
7.38108373553243));
#8515=CARTESIAN_POINT('Ctrl Pts',(-0.211512387655128,-2.8498166397957,7.29998894076038));
#8516=CARTESIAN_POINT('Ctrl Pts',(-0.234672692510252,-2.86193666288461,
7.19851881716116));
#8517=CARTESIAN_POINT('Ctrl Pts',(-0.211502078818359,-2.87409363541626,
7.09651570260184));
#8518=CARTESIAN_POINT('Ctrl Pts',(-0.146175031667225,-2.88628349462379,
7.01496045942807));
#8519=CARTESIAN_POINT('Ctrl Pts',(-0.0201759406699065,-2.90257490033143,
6.95334279019282));
#8520=CARTESIAN_POINT('Ctrl Pts',(0.164048433167981,-2.92300029227989,6.99488705015939));
#8521=CARTESIAN_POINT('Ctrl Pts',(0.263212640482471,-2.94757377707087,7.20034626829039));
#8522=CARTESIAN_POINT('Ctrl Pts',(0.16413428164115,-2.9721746956776,7.40571604889496));
#8523=CARTESIAN_POINT('Ctrl Pts',(-0.0580809020736254,-2.99676718133414,
7.45651943873815));
#8524=CARTESIAN_POINT('Ctrl Pts',(-0.236127517621773,-3.02131545740765,
7.31427023254914));
#8525=CARTESIAN_POINT('Ctrl Pts',(-0.235623291843773,-3.04374517395574,
7.10674242176483));
#8526=CARTESIAN_POINT('Ctrl Pts',(-0.107269644782094,-3.06405280900675,
6.97972425972366));
#8527=CARTESIAN_POINT('Ctrl Pts',(0.0527757922260713,-3.08225163138773,
6.96159979137369));
#8528=CARTESIAN_POINT('Ctrl Pts',(0.188726377923501,-3.10035885514916,7.04734634676648));
#8529=CARTESIAN_POINT('Ctrl Pts',(0.232341637226282,-3.11536108595312,7.17289318656827));
#8530=CARTESIAN_POINT('Ctrl Pts',(0.215074929637344,-3.12730445561105,7.27290788199928));
#8531=CARTESIAN_POINT('Ctrl Pts',(0.166334604203376,-3.13920694864625,7.3615533699487));
#8532=CARTESIAN_POINT('Ctrl Pts',(0.0552567235661542,-3.1540048293497,7.43128948802867));
#8533=CARTESIAN_POINT('Ctrl Pts',(-0.100043793704833,-3.17162317434127,
7.4135433615447));
#8534=CARTESIAN_POINT('Ctrl Pts',(-0.209398878386583,-3.18909256344761,
7.30384381469642));
#8535=CARTESIAN_POINT('Ctrl Pts',(-0.226357160076232,-3.20640410002376,
7.15124619930781));
#8536=CARTESIAN_POINT('Ctrl Pts',(-0.145244888291477,-3.22354989628281,
7.02263774678675));
#8537=CARTESIAN_POINT('Ctrl Pts',(-0.00307739889558988,-3.24052311289208,
6.9731562179116));
#8538=CARTESIAN_POINT('Ctrl Pts',(0.137388780060693,-3.25731801286151,7.02262233145429));
#8539=CARTESIAN_POINT('Ctrl Pts',(0.215568012201749,-3.27392998789316,7.14745036721));
#8540=CARTESIAN_POINT('Ctrl Pts',(0.199056669422034,-3.29035561704227,7.29224338602279));
#8541=CARTESIAN_POINT('Ctrl Pts',(0.0972442378117872,-3.30659260084323,
7.39359267072072));
#8542=CARTESIAN_POINT('Ctrl Pts',(-0.0606078656788346,-3.32442299860284,
7.41159207397961));
#8543=CARTESIAN_POINT('Ctrl Pts',(-0.174349434794334,-3.34024917344643,
7.3202399790036));
#8544=CARTESIAN_POINT('Ctrl Pts',(-0.200242071600934,-3.35415023112003,
7.20325404432313));
#8545=CARTESIAN_POINT('Ctrl Pts',(-0.18063258547865,-3.36449358017806,7.11681410663695));
#8546=CARTESIAN_POINT('Ctrl Pts',(-0.125490051337178,-3.37475550369447,
7.04788845684967));
#8547=CARTESIAN_POINT('Ctrl Pts',(-0.0466957223057233,-3.38493729013136,
7.00998942647324));
#8548=CARTESIAN_POINT('Ctrl Pts',(0.0401186427931673,-3.39504044724382,
7.01009457046437));
#8549=CARTESIAN_POINT('Ctrl Pts',(0.117713403951327,-3.40506669595631,7.04749596858793));
#8550=CARTESIAN_POINT('Ctrl Pts',(0.170930387597076,-3.41501799177983,7.11440539415709));
#8551=CARTESIAN_POINT('Ctrl Pts',(0.18979238088286,-3.42489648282701,7.1971524208448));
#8552=CARTESIAN_POINT('Ctrl Pts',(0.17093827709221,-3.43470453492267,7.2792766512254));
#8553=CARTESIAN_POINT('Ctrl Pts',(0.123087817102158,-3.44363304446436,7.33923456804198));
#8554=CARTESIAN_POINT('Ctrl Pts',(0.0630389653927126,-3.45170235370222,
7.37229315652779));
#8555=CARTESIAN_POINT('Ctrl Pts',(-0.0177036729288226,-3.46133839204526,
7.38615351281265));
#8556=CARTESIAN_POINT('Ctrl Pts',(-0.11772305137169,-3.47329787855213,7.35109019812551));
#8557=CARTESIAN_POINT('Ctrl Pts',(-0.184714685581635,-3.48752403008714,
7.24410703240861));
#8558=CARTESIAN_POINT('Ctrl Pts',(-0.17053859750796,-3.50163575663314,7.11977423357787));
#8559=CARTESIAN_POINT('Ctrl Pts',(-0.082587996452088,-3.51564730527911,
7.03201669890537));
#8560=CARTESIAN_POINT('Ctrl Pts',(0.0401074098738201,-3.52956782204744,
7.0182572369454));
#8561=CARTESIAN_POINT('Ctrl Pts',(0.144033604536224,-3.54341977713357,7.08377705773452));
#8562=CARTESIAN_POINT('Ctrl Pts',(0.170884312908661,-3.55260377562906,7.16051919899628));
#8563=CARTESIAN_POINT('Ctrl Pts',(0.170889524395514,-3.55720086923049,7.1991469511116));
#8564=CARTESIAN_POINT('',(0.199999521685004,-2.62021022067982,7.20354528529548));
#8565=CARTESIAN_POINT('Origin',(0.2,-2.65,7.2));
#8566=CARTESIAN_POINT('',(0.170889524395514,-3.55720086923049,7.1991469511116));
#8567=CARTESIAN_POINT('Ctrl Pts',(0.199999521685004,-2.62021022067982,7.20354528529548));
#8568=CARTESIAN_POINT('Ctrl Pts',(0.19999343949118,-2.6255753643916,7.24862669087077));
#8569=CARTESIAN_POINT('Ctrl Pts',(0.168615691452697,-2.63634781999191,7.33868016798294));
#8570=CARTESIAN_POINT('Ctrl Pts',(0.0459616996448183,-2.65270477799173,
7.41618164971903));
#8571=CARTESIAN_POINT('Ctrl Pts',(-0.0998469869656992,-2.66924595959392,
7.39996507729611));
#8572=CARTESIAN_POINT('Ctrl Pts',(-0.204936181985623,-2.68597304189578,
7.29527847685269));
#8573=CARTESIAN_POINT('Ctrl Pts',(-0.221986969755699,-2.7028797483455,7.14628505326925));
#8574=CARTESIAN_POINT('Ctrl Pts',(-0.141631327334848,-2.71996166380803,
7.01788664502262));
#8575=CARTESIAN_POINT('Ctrl Pts',(0.00270481241442624,-2.73721192504324,
6.96708134679183));
#8576=CARTESIAN_POINT('Ctrl Pts',(0.143039113459417,-2.75397833948373,7.01603761180454));
#8577=CARTESIAN_POINT('Ctrl Pts',(0.223330027417085,-2.77023316539608,7.13370506584288));
#8578=CARTESIAN_POINT('Ctrl Pts',(0.223609433092684,-2.7859516486779,7.2713911725354));
#8579=CARTESIAN_POINT('Ctrl Pts',(0.152101468687107,-2.80045790761646,7.37648984952004));
#8580=CARTESIAN_POINT('Ctrl Pts',(0.0493840180807327,-2.81371750007274,
7.42583309513969));
#8581=CARTESIAN_POINT('Ctrl Pts',(-0.0535656424988984,-2.82570326133932,
7.42596307871198));
#8582=CARTESIAN_POINT('Ctrl Pts',(-0.146731811694293,-2.83773755003964,
7.38108373553243));
#8583=CARTESIAN_POINT('Ctrl Pts',(-0.211512387655128,-2.8498166397957,7.29998894076038));
#8584=CARTESIAN_POINT('Ctrl Pts',(-0.234672692510252,-2.86193666288461,
7.19851881716116));
#8585=CARTESIAN_POINT('Ctrl Pts',(-0.211502078818359,-2.87409363541626,
7.09651570260184));
#8586=CARTESIAN_POINT('Ctrl Pts',(-0.146175031667225,-2.88628349462379,
7.01496045942807));
#8587=CARTESIAN_POINT('Ctrl Pts',(-0.0201759406699065,-2.90257490033143,
6.95334279019282));
#8588=CARTESIAN_POINT('Ctrl Pts',(0.164048433167981,-2.92300029227989,6.99488705015939));
#8589=CARTESIAN_POINT('Ctrl Pts',(0.263212640482471,-2.94757377707087,7.20034626829039));
#8590=CARTESIAN_POINT('Ctrl Pts',(0.16413428164115,-2.9721746956776,7.40571604889496));
#8591=CARTESIAN_POINT('Ctrl Pts',(-0.0580809020736254,-2.99676718133414,
7.45651943873815));
#8592=CARTESIAN_POINT('Ctrl Pts',(-0.236127517621773,-3.02131545740765,
7.31427023254914));
#8593=CARTESIAN_POINT('Ctrl Pts',(-0.235623291843773,-3.04374517395574,
7.10674242176483));
#8594=CARTESIAN_POINT('Ctrl Pts',(-0.107269644782094,-3.06405280900675,
6.97972425972366));
#8595=CARTESIAN_POINT('Ctrl Pts',(0.0527757922260713,-3.08225163138773,
6.96159979137369));
#8596=CARTESIAN_POINT('Ctrl Pts',(0.188726377923501,-3.10035885514916,7.04734634676648));
#8597=CARTESIAN_POINT('Ctrl Pts',(0.232341637226282,-3.11536108595312,7.17289318656827));
#8598=CARTESIAN_POINT('Ctrl Pts',(0.215074929637344,-3.12730445561105,7.27290788199928));
#8599=CARTESIAN_POINT('Ctrl Pts',(0.166334604203376,-3.13920694864625,7.3615533699487));
#8600=CARTESIAN_POINT('Ctrl Pts',(0.0552567235661542,-3.1540048293497,7.43128948802867));
#8601=CARTESIAN_POINT('Ctrl Pts',(-0.100043793704833,-3.17162317434127,
7.4135433615447));
#8602=CARTESIAN_POINT('Ctrl Pts',(-0.209398878386583,-3.18909256344761,
7.30384381469642));
#8603=CARTESIAN_POINT('Ctrl Pts',(-0.226357160076232,-3.20640410002376,
7.15124619930781));
#8604=CARTESIAN_POINT('Ctrl Pts',(-0.145244888291477,-3.22354989628281,
7.02263774678675));
#8605=CARTESIAN_POINT('Ctrl Pts',(-0.00307739889558988,-3.24052311289208,
6.9731562179116));
#8606=CARTESIAN_POINT('Ctrl Pts',(0.137388780060693,-3.25731801286151,7.02262233145429));
#8607=CARTESIAN_POINT('Ctrl Pts',(0.215568012201749,-3.27392998789316,7.14745036721));
#8608=CARTESIAN_POINT('Ctrl Pts',(0.199056669422034,-3.29035561704227,7.29224338602279));
#8609=CARTESIAN_POINT('Ctrl Pts',(0.0972442378117872,-3.30659260084323,
7.39359267072072));
#8610=CARTESIAN_POINT('Ctrl Pts',(-0.0606078656788346,-3.32442299860284,
7.41159207397961));
#8611=CARTESIAN_POINT('Ctrl Pts',(-0.174349434794334,-3.34024917344643,
7.3202399790036));
#8612=CARTESIAN_POINT('Ctrl Pts',(-0.200242071600934,-3.35415023112003,
7.20325404432313));
#8613=CARTESIAN_POINT('Ctrl Pts',(-0.18063258547865,-3.36449358017806,7.11681410663695));
#8614=CARTESIAN_POINT('Ctrl Pts',(-0.125490051337178,-3.37475550369447,
7.04788845684967));
#8615=CARTESIAN_POINT('Ctrl Pts',(-0.0466957223057233,-3.38493729013136,
7.00998942647324));
#8616=CARTESIAN_POINT('Ctrl Pts',(0.0401186427931673,-3.39504044724382,
7.01009457046437));
#8617=CARTESIAN_POINT('Ctrl Pts',(0.117713403951327,-3.40506669595631,7.04749596858793));
#8618=CARTESIAN_POINT('Ctrl Pts',(0.170930387597076,-3.41501799177983,7.11440539415709));
#8619=CARTESIAN_POINT('Ctrl Pts',(0.18979238088286,-3.42489648282701,7.1971524208448));
#8620=CARTESIAN_POINT('Ctrl Pts',(0.17093827709221,-3.43470453492267,7.2792766512254));
#8621=CARTESIAN_POINT('Ctrl Pts',(0.123087817102158,-3.44363304446436,7.33923456804198));
#8622=CARTESIAN_POINT('Ctrl Pts',(0.0630389653927126,-3.45170235370222,
7.37229315652779));
#8623=CARTESIAN_POINT('Ctrl Pts',(-0.0177036729288226,-3.46133839204526,
7.38615351281265));
#8624=CARTESIAN_POINT('Ctrl Pts',(-0.11772305137169,-3.47329787855213,7.35109019812551));
#8625=CARTESIAN_POINT('Ctrl Pts',(-0.184714685581635,-3.48752403008714,
7.24410703240861));
#8626=CARTESIAN_POINT('Ctrl Pts',(-0.17053859750796,-3.50163575663314,7.11977423357787));
#8627=CARTESIAN_POINT('Ctrl Pts',(-0.082587996452088,-3.51564730527911,
7.03201669890537));
#8628=CARTESIAN_POINT('Ctrl Pts',(0.0401074098738201,-3.52956782204744,
7.0182572369454));
#8629=CARTESIAN_POINT('Ctrl Pts',(0.144033604536224,-3.54341977713357,7.08377705773452));
#8630=CARTESIAN_POINT('Ctrl Pts',(0.170884312908661,-3.55260377562906,7.16051919899628));
#8631=CARTESIAN_POINT('Ctrl Pts',(0.170889524395514,-3.55720086923049,7.1991469511116));
#8632=CARTESIAN_POINT('Origin',(0.2,-3.55,7.2));
#8633=CARTESIAN_POINT('Origin',(0.2,-3.55,7.2));
#8634=CARTESIAN_POINT('Origin',(0.2,-2.65,7.2));
#9758=UNCERTAINTY_MEASURE_WITH_UNIT(LENGTH_MEASURE(0.001),#9814,
'DISTANCE_ACCURACY_VALUE',
'Maximum model space distance between geometric entities at asserted c
onnectivities');
#9777=UNCERTAINTY_MEASURE_WITH_UNIT(LENGTH_MEASURE(0.001),#9814,
'DISTANCE_ACCURACY_VALUE',
'Maximum model space distance between geometric entities at asserted c
onnectivities');
#9794=(
GEOMETRIC_REPRESENTATION_CONTEXT(3)
GLOBAL_UNCERTAINTY_ASSIGNED_CONTEXT((#9758))
GLOBAL_UNIT_ASSIGNED_CONTEXT((#9814,#9816,#9817))
REPRESENTATION_CONTEXT('','3D')
);
#9813=(
GEOMETRIC_REPRESENTATION_CONTEXT(3)
GLOBAL_UNCERTAINTY_ASSIGNED_CONTEXT((#9777))
GLOBAL_UNIT_ASSIGNED_CONTEXT((#9814,#9816,#9817))
REPRESENTATION_CONTEXT('','3D')
);
#9814=(
LENGTH_UNIT()
NAMED_UNIT(*)
SI_UNIT(.CENTI.,.METRE.)
);
#9816=(
NAMED_UNIT(*)
PLANE_ANGLE_UNIT()
SI_UNIT($,.RADIAN.)
);
#9817=(
NAMED_UNIT(*)
SI_UNIT($,.STERADIAN.)
SOLID_ANGLE_UNIT()
);
#9834=SHAPE_DEFINITION_REPRESENTATION(#9869,#9951);
#9869=PRODUCT_DEFINITION_SHAPE('',$,#9987);
#9951=SHAPE_REPRESENTATION('',(#5390),#9794);
#9970=PRODUCT_DEFINITION_CONTEXT('part definition',#10077,'design');
#9987=PRODUCT_DEFINITION('Detent spring','Detent spring',#10022,#9970);
#10022=PRODUCT_DEFINITION_FORMATION('',$,#10095);
#10077=APPLICATION_CONTEXT(
'Core Data for Automotive Mechanical Design Process');
#10078=PRODUCT_CONTEXT('part definition',#10077,'mechanical');
#10095=PRODUCT('Detent spring','Detent spring','Detent spring',(#10078));
#10177=COLOUR_RGB('Grey',0.48,0.52,0.57);
#10178=FILL_AREA_STYLE_COLOUR('',#10177);
#10179=FILL_AREA_STYLE('',(#10178));
#10180=SURFACE_STYLE_FILL_AREA(#10179);
#10181=SURFACE_SIDE_STYLE('',(#10180));
#10182=SURFACE_STYLE_USAGE(.BOTH.,#10181);
#10183=PRESENTATION_STYLE_ASSIGNMENT((#10182));
ENDSEC;
END-ISO-10303-21;
